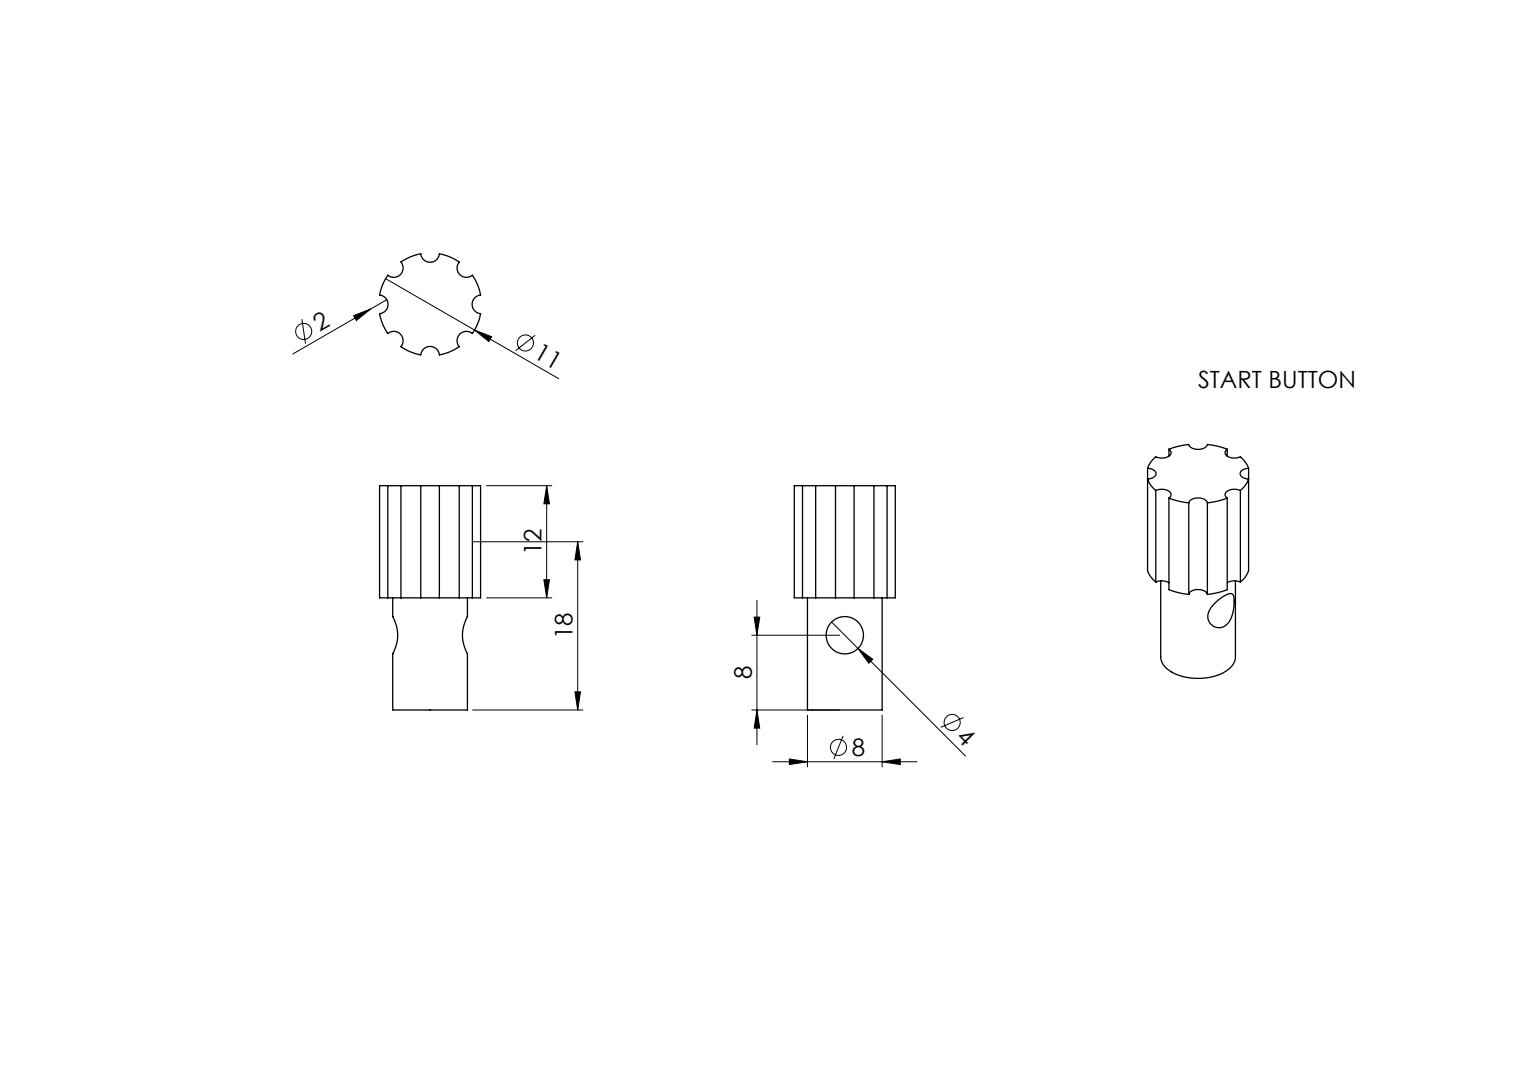
ISO-10303-21;
HEADER;
FILE_DESCRIPTION (('STEP AP214'),
    '1' );
FILE_NAME ('start button.step',
    '2026-10-26T11:20:31',
    ( '' ),
    ( '' ),
    'SwSTEP 2.0',
    'SolidWorks 2026',
    '' );
FILE_SCHEMA (( 'AUTOMOTIVE_DESIGN' ));
ENDSEC;

DATA;
#3=ORIENTED_EDGE ( 'NONE', *, *, #2058, .T. ) ;
#5=DIRECTION ( 'NONE',  ( 0.000000000000000000, 0.000000000000000000, 1.000000000000000000 ) ) ;
#6=ORIENTED_EDGE ( 'NONE', *, *, #2251, .T. ) ;
#8=ORIENTED_EDGE ( 'NONE', *, *, #613, .T. ) ;
#11=CARTESIAN_POINT ( 'NONE',  ( 3.575465955037824273, 33.89312899261130951, 7.205771075917312807 ) ) ;
#13=CARTESIAN_POINT ( 'NONE',  ( 3.900351855253538336, 31.20702153671021861, 9.895868398202676275 ) ) ;
#16=AXIS2_PLACEMENT_3D ( 'NONE', #2193, #1531, #438 ) ;
#20=AXIS2_PLACEMENT_3D ( 'NONE', #4406, #1830, #790 ) ;
#21=ORIENTED_EDGE ( 'NONE', *, *, #745, .T. ) ;
#25=CARTESIAN_POINT ( 'NONE',  ( -3.889087296526001047, 37.00000000000000000, 5.110912703473974084 ) ) ;
#26=DIRECTION ( 'NONE',  ( 0.000000000000000000, 0.000000000000000000, -1.000000000000000000 ) ) ;
#28=ORIENTED_EDGE ( 'NONE', *, *, #250, .F. ) ;
#35=APPLICATION_CONTEXT ( 'automotive_design' ) ;
#47=CARTESIAN_POINT ( 'NONE',  ( -3.606497132222527213, 31.99144327829980838, 10.73188315364928691 ) ) ;
#50=EDGE_CURVE ( 'NONE', #1185, #1168, #2904, .T. ) ;
#51=ORIENTED_EDGE ( 'NONE', *, *, #696, .F. ) ;
#52=VERTEX_POINT ( 'NONE', #2322 ) ;
#53=ORIENTED_EDGE ( 'NONE', *, *, #2142, .T. ) ;
#55=CIRCLE ( 'NONE', #1867, 1.000000000000000000 ) ;
#61=CARTESIAN_POINT ( 'NONE',  ( 3.120626071653185285, 37.00000000000000000, 4.471016347907789346 ) ) ;
#63=CIRCLE ( 'NONE', #1740, 4.000000000000000000 ) ;
#68=ADVANCED_FACE ( 'NONE', ( #4153 ), #1596, .T. ) ;
#73=CARTESIAN_POINT ( 'NONE',  ( -3.522877905629562711, 32.34829198493223146, 10.89542184998092367 ) ) ;
#76=EDGE_LOOP ( 'NONE', ( #1998, #356, #1571, #3856 ) ) ;
#84=EDGE_CURVE ( 'NONE', #2338, #1148, #4563, .T. ) ;
#86=EDGE_CURVE ( 'NONE', #3119, #3855, #2573, .T. ) ;
#94=LINE ( 'NONE', #3342, #4161 ) ;
#98=DIRECTION ( 'NONE',  ( 0.000000000000000000, 0.000000000000000000, 1.000000000000000000 ) ) ;
#103=EDGE_LOOP ( 'NONE', ( #598, #2944, #3052, #880 ) ) ;
#104=ORIENTED_EDGE ( 'NONE', *, *, #1011, .F. ) ;
#106=CARTESIAN_POINT ( 'NONE',  ( -3.889087296526001047, 37.00000000000000000, 5.110912703473974084 ) ) ;
#109=ORIENTED_EDGE ( 'NONE', *, *, #4683, .T. ) ;
#114=CARTESIAN_POINT ( 'NONE',  ( 2.255140518769849223E-14, 37.00000000000000000, 4.499999999999992895 ) ) ;
#116=CARTESIAN_POINT ( 'NONE',  ( -4.000043395258027878, 35.00008679053002680, 9.131973577465634762 ) ) ;
#120=CARTESIAN_POINT ( 'NONE',  ( 3.469446951953614189E-15, 37.00000000000000000, 8.999999999999992895 ) ) ;
#129=( GEOMETRIC_REPRESENTATION_CONTEXT ( 3 ) GLOBAL_UNCERTAINTY_ASSIGNED_CONTEXT ( ( #2638 ) ) GLOBAL_UNIT_ASSIGNED_CONTEXT ( ( #3790, #2760, #4527 ) ) REPRESENTATION_CONTEXT ( 'NONE', 'WORKASPACE' ) );
#133=DIRECTION ( 'NONE',  ( 0.000000000000000000, 0.000000000000000000, 1.000000000000000000 ) ) ;
#134=ORIENTED_EDGE ( 'NONE', *, *, #2569, .F. ) ;
#139=CARTESIAN_POINT ( 'NONE',  ( 2.255140518769849223E-14, 37.00000000000000000, 3.499999999999992895 ) ) ;
#141=CARTESIAN_POINT ( 'NONE',  ( -5.409090909090905619, 33.00000000000000000, 6.999999999999991118 ) ) ;
#145=CARTESIAN_POINT ( 'NONE',  ( 3.809567799457752368, 34.58652683892340463, 10.22463024623739081 ) ) ;
#154=SURFACE_STYLE_FILL_AREA ( #887 ) ;
#156=DIRECTION ( 'NONE',  ( 0.000000000000000000, 0.000000000000000000, 1.000000000000000000 ) ) ;
#158=DIRECTION ( 'NONE',  ( -0.000000000000000000, -1.000000000000000000, -0.000000000000000000 ) ) ;
#159=CARTESIAN_POINT ( 'NONE',  ( 3.120626071653123113, 37.00000000000000000, 13.52898365209223996 ) ) ;
#160=ORIENTED_EDGE ( 'NONE', *, *, #4437, .T. ) ;
#165=CARTESIAN_POINT ( 'NONE',  ( 3.967498225428659264, 34.93431228236265440, 8.474567154859101947 ) ) ;
#172=EDGE_LOOP ( 'NONE', ( #4370, #2757, #3708, #3979 ) ) ;
#178=LINE ( 'NONE', #2303, #3205 ) ;
#182=FACE_OUTER_BOUND ( 'NONE', #1092, .T. ) ;
#188=ORIENTED_EDGE ( 'NONE', *, *, #4683, .F. ) ;
#203=CARTESIAN_POINT ( 'NONE',  ( -3.889087296526055226, 49.00000000000000000, 12.88908729652595753 ) ) ;
#210=CARTESIAN_POINT ( 'NONE',  ( -3.464101615137750390, 33.00000000000000000, 6.999999999999991118 ) ) ;
#213=VERTEX_POINT ( 'NONE', #2094 ) ;
#215=EDGE_CURVE ( 'NONE', #3697, #378, #1086, .T. ) ;
#222=AXIS2_PLACEMENT_3D ( 'NONE', #601, #2758, #3141 ) ;
#223=ORIENTED_EDGE ( 'NONE', *, *, #3395, .T. ) ;
#231=CARTESIAN_POINT ( 'NONE',  ( -3.889087296526001047, 34.17157287525380838, 5.110912703473974084 ) ) ;
#233=VECTOR ( 'NONE', #4216, 1000.000000000000000 ) ;
#237=ORIENTED_EDGE ( 'NONE', *, *, #1871, .T. ) ;
#243=CIRCLE ( 'NONE', #3040, 1.000000000000000000 ) ;
#250=EDGE_CURVE ( 'NONE', #1339, #1902, #257, .T. ) ;
#253=EDGE_CURVE ( 'NONE', #1148, #1902, #1067, .T. ) ;
#257=LINE ( 'NONE', #3875, #233 ) ;
#264=AXIS2_PLACEMENT_3D ( 'NONE', #4299, #3243, #659 ) ;
#267=ADVANCED_FACE ( 'NONE', ( #621 ), #905, .F. ) ;
#269=DIRECTION ( 'NONE',  ( -0.000000000000000000, -1.000000000000000000, -0.000000000000000000 ) ) ;
#273=DIRECTION ( 'NONE',  ( 0.000000000000000000, 1.000000000000000000, 0.000000000000000000 ) ) ;
#277=VECTOR ( 'NONE', #1465, 1000.000000000000000 ) ;
#286=CARTESIAN_POINT ( 'NONE',  ( 3.469446951953614189E-15, 49.00000000000000000, 8.999999999999992895 ) ) ;
#291=AXIS2_PLACEMENT_3D ( 'NONE', #4539, #997, #2087 ) ;
#293=CARTESIAN_POINT ( 'NONE',  ( -3.120626071653146649, 43.00000000000000000, 4.471016347907768029 ) ) ;
#294=CIRCLE ( 'NONE', #1500, 1.000000000000000000 ) ;
#304=ORIENTED_EDGE ( 'NONE', *, *, #711, .T. ) ;
#306=CARTESIAN_POINT ( 'NONE',  ( 5.500000000000003553, 34.17157287525380838, 8.999999999999992895 ) ) ;
#307=VECTOR ( 'NONE', #4096, 1000.000000000000000 ) ;
#319=CARTESIAN_POINT ( 'NONE',  ( 3.993269581196953411, 31.01336414471273883, 8.733908321742495318 ) ) ;
#335=APPLICATION_CONTEXT ( 'automotive_design' ) ;
#341=DIRECTION ( 'NONE',  ( 1.000000000000000000, -0.000000000000000000, -0.000000000000000000 ) ) ;
#342=VECTOR ( 'NONE', #432, 1000.000000000000000 ) ;
#345=MECHANICAL_DESIGN_GEOMETRIC_PRESENTATION_REPRESENTATION('',(#2384),#129);
#356=ORIENTED_EDGE ( 'NONE', *, *, #4437, .F. ) ;
#358=CARTESIAN_POINT ( 'NONE',  ( 3.999885695961631793, 34.99977139185988051, 9.266511461428612151 ) ) ;
#359=CARTESIAN_POINT ( 'NONE',  ( -5.409090909090905619, 43.00000000000000000, 9.995859195463930646 ) ) ;
#361=CARTESIAN_POINT ( 'NONE',  ( 3.464101615137758383, 32.86534535152231484, 6.999999999999992006 ) ) ;
#366=CARTESIAN_POINT ( 'NONE',  ( 4.528983652092195555, 37.00000000000000000, 12.12062607165318973 ) ) ;
#367=AXIS2_PLACEMENT_3D ( 'NONE', #1611, #4592, #2382 ) ;
#371=ORIENTED_EDGE ( 'NONE', *, *, #2152, .T. ) ;
#377=VERTEX_POINT ( 'NONE', #3443 ) ;
#378=VERTEX_POINT ( 'NONE', #2133 ) ;
#391=CARTESIAN_POINT ( 'NONE',  ( -3.967441838779837582, 34.93419588968778555, 9.525690396061339271 ) ) ;
#393=VECTOR ( 'NONE', #632, 1000.000000000000000 ) ;
#395=EDGE_LOOP ( 'NONE', ( #4328, #2140, #4671, #3538 ) ) ;
#408=ORIENTED_EDGE ( 'NONE', *, *, #542, .F. ) ;
#411=CARTESIAN_POINT ( 'NONE',  ( 3.522982843720159796, 32.34803768106982602, 10.89519766348715102 ) ) ;
#412=CIRCLE ( 'NONE', #3674, 1.000000000000000000 ) ;
#415=CARTESIAN_POINT ( 'NONE',  ( -3.889087296526001047, 49.00000000000000000, 6.110912703473974084 ) ) ;
#432=DIRECTION ( 'NONE',  ( 0.000000000000000000, -1.000000000000000000, 0.000000000000000000 ) ) ;
#438=DIRECTION ( 'NONE',  ( 0.000000000000000000, 0.000000000000000000, 1.000000000000000000 ) ) ;
#439=CARTESIAN_POINT ( 'NONE',  ( -5.499999999999996447, 34.17157287525380838, 8.999999999999992895 ) ) ;
#441=CARTESIAN_POINT ( 'NONE',  ( -3.672134815396410179, 34.23001392835894308, 10.59780778022629377 ) ) ;
#445=CARTESIAN_POINT ( 'NONE',  ( -3.501495480098614443, 32.47366590808272235, 10.93402018205975601 ) ) ;
#446=CARTESIAN_POINT ( 'NONE',  ( 3.469446951953614189E-15, 49.00000000000000000, 8.999999999999992895 ) ) ;
#448=CARTESIAN_POINT ( 'NONE',  ( 3.469446951953614189E-15, 49.00000000000000000, 8.999999999999992895 ) ) ;
#451=AXIS2_PLACEMENT_3D ( 'NONE', #3078, #2717, #4317 ) ;
#460=VERTEX_POINT ( 'NONE', #3272 ) ;
#468=VERTEX_POINT ( 'NONE', #4017 ) ;
#479=DIRECTION ( 'NONE',  ( 0.000000000000000000, 1.000000000000000000, 0.000000000000000000 ) ) ;
#486=CARTESIAN_POINT ( 'NONE',  ( 3.601048973789312324, 31.98899025511026650, 10.74504312029988284 ) ) ;
#487=PRODUCT_DEFINITION ( 'UNKNOWN', '', #1349, #2416 ) ;
#494=CARTESIAN_POINT ( 'NONE',  ( 3.971780439164239063, 34.94497680528392891, 9.533653685786569909 ) ) ;
#497=DIRECTION ( 'NONE',  ( 0.000000000000000000, 0.000000000000000000, 1.000000000000000000 ) ) ;
#502=CARTESIAN_POINT ( 'NONE',  ( -3.120626071653146649, 49.00000000000000000, 4.471016347907768029 ) ) ;
#504=CARTESIAN_POINT ( 'NONE',  ( 4.528983652092238188, 37.00000000000000000, 5.879373928346857348 ) ) ;
#507=PRODUCT ( 'start button', 'start button', '', ( #1061 ) ) ;
#515=CARTESIAN_POINT ( 'NONE',  ( -3.889087296526001047, 34.17157287525380838, 6.110912703473974084 ) ) ;
#523=DIRECTION ( 'NONE',  ( 0.000000000000000000, 1.000000000000000000, -0.000000000000000000 ) ) ;
#525=VERTEX_POINT ( 'NONE', #3971 ) ;
#528=ORIENTED_EDGE ( 'NONE', *, *, #2213, .T. ) ;
#530=FACE_OUTER_BOUND ( 'NONE', #2627, .T. ) ;
#538=EDGE_CURVE ( 'NONE', #3343, #4108, #2239, .T. ) ;
#542=EDGE_CURVE ( 'NONE', #3343, #1490, #1089, .T. ) ;
#543=EDGE_CURVE ( 'NONE', #1651, #1279, #3319, .T. ) ;
#551=ORIENTED_EDGE ( 'NONE', *, *, #253, .F. ) ;
#558=CARTESIAN_POINT ( 'NONE',  ( 0.9958591954638854604, 37.00000000000000000, 14.40909090909091184 ) ) ;
#559=CARTESIAN_POINT ( 'NONE',  ( -4.528983652092210654, 49.00000000000000000, 5.879373928346826261 ) ) ;
#560=CARTESIAN_POINT ( 'NONE',  ( 5.409090909090911836, 37.00000000000000000, 8.004140804536053366 ) ) ;
#564=EDGE_CURVE ( 'NONE', #213, #2091, #3689, .T. ) ;
#565=CARTESIAN_POINT ( 'NONE',  ( 0.9958591954638856825, 49.00000000000000000, 14.40909090909091361 ) ) ;
#573=ORIENTED_EDGE ( 'NONE', *, *, #86, .F. ) ;
#574=VERTEX_POINT ( 'NONE', #3294 ) ;
#577=DIRECTION ( 'NONE',  ( 0.000000000000000000, 0.000000000000000000, -1.000000000000000000 ) ) ;
#581=DIRECTION ( 'NONE',  ( 0.000000000000000000, 0.000000000000000000, -1.000000000000000000 ) ) ;
#583=EDGE_CURVE ( 'NONE', #763, #2091, #94, .T. ) ;
#589=VECTOR ( 'NONE', #847, 1000.000000000000000 ) ;
#597=CARTESIAN_POINT ( 'NONE',  ( 3.889087296526035242, 49.00000000000000000, 5.110912703473999841 ) ) ;
#598=ORIENTED_EDGE ( 'NONE', *, *, #3273, .T. ) ;
#599=EDGE_LOOP ( 'NONE', ( #237, #2178, #2583, #28 ) ) ;
#601=CARTESIAN_POINT ( 'NONE',  ( 3.469446951953614189E-15, 49.00000000000000000, 8.999999999999992895 ) ) ;
#604=( NAMED_UNIT ( * ) SI_UNIT ( $, .STERADIAN. ) SOLID_ANGLE_UNIT ( ) );
#605=DIRECTION ( 'NONE',  ( -0.000000000000000000, 1.000000000000000000, -0.000000000000000000 ) ) ;
#608=LINE ( 'NONE', #3479, #393 ) ;
#610=DIRECTION ( 'NONE',  ( 0.000000000000000000, 0.000000000000000000, 1.000000000000000000 ) ) ;
#613=EDGE_CURVE ( 'NONE', #1651, #574, #4113, .T. ) ;
#621=FACE_OUTER_BOUND ( 'NONE', #395, .T. ) ;
#626=CARTESIAN_POINT ( 'NONE',  ( -0.9958591954639161026, 37.00000000000000000, 3.590909090909080170 ) ) ;
#628=DIRECTION ( 'NONE',  ( 0.000000000000000000, 0.000000000000000000, 1.000000000000000000 ) ) ;
#631=CIRCLE ( 'NONE', #2748, 5.500000000000000000 ) ;
#632=DIRECTION ( 'NONE',  ( -0.000000000000000000, 1.000000000000000000, -0.000000000000000000 ) ) ;
#646=ORIENTED_EDGE ( 'NONE', *, *, #4119, .F. ) ;
#653=CARTESIAN_POINT ( 'NONE',  ( 3.959305671612554781E-15, 43.00000000000000000, 12.99999999999999289 ) ) ;
#659=DIRECTION ( 'NONE',  ( 0.000000000000000000, -0.000000000000000000, 1.000000000000000000 ) ) ;
#666=CARTESIAN_POINT ( 'NONE',  ( -3.889087296526055226, 34.17157287525380838, 12.88908729652595753 ) ) ;
#670=FACE_OUTER_BOUND ( 'NONE', #858, .T. ) ;
#671=DIRECTION ( 'NONE',  ( -0.000000000000000000, -1.000000000000000000, -0.000000000000000000 ) ) ;
#675=ORIENTED_EDGE ( 'NONE', *, *, #4119, .T. ) ;
#683=CARTESIAN_POINT ( 'NONE',  ( 3.809991693235077026, 31.40492942523385267, 7.766500207085086593 ) ) ;
#692=AXIS2_PLACEMENT_3D ( 'NONE', #597, #3115, #4195 ) ;
#696=EDGE_CURVE ( 'NONE', #4356, #1339, #886, .T. ) ;
#709=FACE_BOUND ( 'NONE', #2678, .T. ) ;
#711=EDGE_CURVE ( 'NONE', #3855, #2686, #2311, .T. ) ;
#717=CARTESIAN_POINT ( 'NONE',  ( -5.409090909090905619, 33.00000000000000000, 10.99999999999999289 ) ) ;
#734=CARTESIAN_POINT ( 'NONE',  ( -3.523144759583856978, 33.65295909972188326, 7.105089090000585195 ) ) ;
#738=CARTESIAN_POINT ( 'NONE',  ( -3.575465955037816723, 32.10687100738867628, 7.205771075917310142 ) ) ;
#743=ORIENTED_EDGE ( 'NONE', *, *, #50, .F. ) ;
#745=EDGE_CURVE ( 'NONE', #378, #1543, #4609, .T. ) ;
#752=CARTESIAN_POINT ( 'NONE',  ( 3.501320667853366153, 32.47456368659583603, 10.93433813232663887 ) ) ;
#760=DIRECTION ( 'NONE',  ( 0.000000000000000000, 0.000000000000000000, 1.000000000000000000 ) ) ;
#763=VERTEX_POINT ( 'NONE', #565 ) ;
#764=ORIENTED_EDGE ( 'NONE', *, *, #2794, .T. ) ;
#782=CIRCLE ( 'NONE', #2359, 5.500000000000000000 ) ;
#783=ORIENTED_EDGE ( 'NONE', *, *, #925, .T. ) ;
#785=CARTESIAN_POINT ( 'NONE',  ( -3.706735793540070656, 31.67823920415836625, 7.493470964888215846 ) ) ;
#790=DIRECTION ( 'NONE',  ( 0.000000000000000000, -0.000000000000000000, 1.000000000000000000 ) ) ;
#801=DIRECTION ( 'NONE',  ( -0.000000000000000000, -1.000000000000000000, -0.000000000000000000 ) ) ;
#806=FACE_OUTER_BOUND ( 'NONE', #1194, .T. ) ;
#810=ORIENTED_EDGE ( 'NONE', *, *, #1129, .F. ) ;
#813=CARTESIAN_POINT ( 'NONE',  ( -5.409090909090905619, 33.00000000000000000, 8.999999999999992895 ) ) ;
#816=VERTEX_POINT ( 'NONE', #949 ) ;
#825=CARTESIAN_POINT ( 'NONE',  ( -3.775090262067420710, 34.50279623606592594, 10.32592777499123748 ) ) ;
#834=VERTEX_POINT ( 'NONE', #3943 ) ;
#842=EDGE_LOOP ( 'NONE', ( #3173, #371, #223, #2579 ) ) ;
#844=DIRECTION ( 'NONE',  ( 0.000000000000000000, -1.000000000000000000, 0.000000000000000000 ) ) ;
#845=CARTESIAN_POINT ( 'NONE',  ( 3.464101615137758827, 32.86736921533707800, 10.99999999999999822 ) ) ;
#847=DIRECTION ( 'NONE',  ( 1.000000000000000000, -0.000000000000000000, -0.000000000000000000 ) ) ;
#851=CARTESIAN_POINT ( 'NONE',  ( -3.889087296526001047, 37.00000000000000000, 6.110912703473974084 ) ) ;
#852=AXIS2_PLACEMENT_3D ( 'NONE', #4182, #2344, #156 ) ;
#854=CARTESIAN_POINT ( 'NONE',  ( 3.120626071653123557, 49.00000000000000000, 13.52898365209223996 ) ) ;
#857=EDGE_LOOP ( 'NONE', ( #3821, #3714, #2924, #2649 ) ) ;
#858=EDGE_LOOP ( 'NONE', ( #109, #134, #2567, #1803 ) ) ;
#870=AXIS2_PLACEMENT_3D ( 'NONE', #231, #973, #4564 ) ;
#872=VECTOR ( 'NONE', #2620, 1000.000000000000000 ) ;
#873=DIRECTION ( 'NONE',  ( -0.000000000000000000, 1.000000000000000000, -0.000000000000000000 ) ) ;
#874=CARTESIAN_POINT ( 'NONE',  ( 2.255140518769849223E-14, 49.00000000000000000, 3.499999999999992895 ) ) ;
#876=CARTESIAN_POINT ( 'NONE',  ( 3.672066530599467971, 34.22247196340288866, 10.58813356411693185 ) ) ;
#880=ORIENTED_EDGE ( 'NONE', *, *, #583, .T. ) ;
#881=ORIENTED_EDGE ( 'NONE', *, *, #3334, .F. ) ;
#886=CIRCLE ( 'NONE', #3466, 5.500000000000000000 ) ;
#887=FILL_AREA_STYLE ('',( #1690 ) ) ;
#889=CARTESIAN_POINT ( 'NONE',  ( 3.889087296526035242, 49.00000000000000000, 5.110912703473999841 ) ) ;
#905=CYLINDRICAL_SURFACE ( 'NONE', #367, 1.000000000000000000 ) ;
#917=( LENGTH_UNIT ( ) NAMED_UNIT ( * ) SI_UNIT ( .MILLI., .METRE. ) );
#922=CARTESIAN_POINT ( 'NONE',  ( -5.409090909090905619, 49.00000000000000000, 9.995859195463930646 ) ) ;
#924=EDGE_CURVE ( 'NONE', #816, #2965, #55, .T. ) ;
#925=EDGE_CURVE ( 'NONE', #1922, #378, #3566, .T. ) ;
#926=DIRECTION ( 'NONE',  ( 0.000000000000000000, 0.000000000000000000, -1.000000000000000000 ) ) ;
#934=ORIENTED_EDGE ( 'NONE', *, *, #3848, .F. ) ;
#936=DIRECTION ( 'NONE',  ( 0.000000000000000000, 1.000000000000000000, 0.000000000000000000 ) ) ;
#938=FACE_OUTER_BOUND ( 'NONE', #842, .T. ) ;
#939=B_SPLINE_CURVE_WITH_KNOTS ( 'NONE', 3,
 ( #3550, #361, #4320, #3942, #4662, #2626, #1434, #683, #1814, #2127, #1391, #319, #1769, #3219, #4687, #1060, #3265, #13, #1456, #1108, #3645, #2237, #486, #411, #752, #3006, #845, #4435 ),
 .UNSPECIFIED., .F., .F.,
 ( 4, 2, 2, 2, 2, 2, 2, 2, 2, 2, 2, 2, 2, 4 ),
 ( 0.000000000000000000, 0.0003975746136738169344, 0.0007951492273476338688, 0.001590298454695268605, 0.002385447682042902799, 0.002783022295716720655, 0.003180596909390538511, 0.003578171523064356367, 0.003975746136738174223, 0.004373320750411992079, 0.004770895364085809068, 0.005566044591433457790, 0.005963619205107282585, 0.006361193818781106513 ),
 .UNSPECIFIED. ) ;
#940=FACE_OUTER_BOUND ( 'NONE', #970, .T. ) ;
#941=VECTOR ( 'NONE', #269, 1000.000000000000000 ) ;
#942=ORIENTED_EDGE ( 'NONE', *, *, #2058, .F. ) ;
#949=CARTESIAN_POINT ( 'NONE',  ( 3.889087296526035242, 37.00000000000000000, 6.110912703473999841 ) ) ;
#961=CYLINDRICAL_SURFACE ( 'NONE', #2888, 5.500000000000000000 ) ;
#963=B_SPLINE_CURVE_WITH_KNOTS ( 'NONE', 3,
 ( #3619, #2631, #2268, #2675, #1974, #1608, #1899, #876, #2247, #4140, #145, #2313, #4359, #494, #358, #3781, #1585, #165, #2291, #3061, #4516, #1103, #3983, #1809, #11, #1451, #1949, #4094, #3370, #2907 ),
 .UNSPECIFIED., .F., .F.,
 ( 4, 2, 2, 2, 2, 2, 2, 2, 2, 2, 2, 2, 2, 2, 4 ),
 ( 0.006361193818781106513, 0.006758065648931968657, 0.007154937479082830801, 0.007551809309233692945, 0.007948681139384555089, 0.008345552969535416366, 0.008742424799686279377, 0.009536168459987998461, 0.009933040290138858003, 0.01032991212028971928, 0.01112365578059143836, 0.01152052761074228923, 0.01191739944089314357, 0.01231427127104399617, 0.01271114310119484878 ),
 .UNSPECIFIED. ) ;
#964=FACE_OUTER_BOUND ( 'NONE', #1217, .T. ) ;
#967=( NAMED_UNIT ( * ) PLANE_ANGLE_UNIT ( ) SI_UNIT ( $, .RADIAN. ) );
#970=EDGE_LOOP ( 'NONE', ( #3118, #2045, #646, #4146 ) ) ;
#973=DIRECTION ( 'NONE',  ( -0.000000000000000000, 1.000000000000000000, -0.000000000000000000 ) ) ;
#986=DIRECTION ( 'NONE',  ( 0.000000000000000000, 1.000000000000000000, 0.000000000000000000 ) ) ;
#997=DIRECTION ( 'NONE',  ( 0.000000000000000000, 1.000000000000000000, 0.000000000000000000 ) ) ;
#1007=DIRECTION ( 'NONE',  ( 0.000000000000000000, 0.000000000000000000, 1.000000000000000000 ) ) ;
#1011=EDGE_CURVE ( 'NONE', #1930, #2608, #4613, .T. ) ;
#1012=ADVANCED_FACE ( 'NONE', ( #1758, #3611 ), #1380, .T. ) ;
#1013=DIRECTION ( 'NONE',  ( 0.000000000000000000, 0.000000000000000000, 1.000000000000000000 ) ) ;
#1019=CARTESIAN_POINT ( 'NONE',  ( -3.967457472430134580, 34.93422823600056404, 8.474369013652145455 ) ) ;
#1022=CIRCLE ( 'NONE', #1936, 1.000000000000000888 ) ;
#1044=CARTESIAN_POINT ( 'NONE',  ( 3.469446951953614189E-15, 43.00000000000000000, 8.999999999999992895 ) ) ;
#1051=CARTESIAN_POINT ( 'NONE',  ( 2.255140518769849223E-14, 34.17157287525380838, 4.499999999999992895 ) ) ;
#1056=CARTESIAN_POINT ( 'NONE',  ( 3.469446951953614189E-15, 37.00000000000000000, 8.999999999999992895 ) ) ;
#1060=CARTESIAN_POINT ( 'NONE',  ( 3.967441838779844687, 31.06580411031222866, 9.525690396061342824 ) ) ;
#1061=PRODUCT_CONTEXT ( 'NONE', #335, 'mechanical' ) ;
#1066=EDGE_CURVE ( 'NONE', #3374, #1168, #4164, .T. ) ;
#1067=CIRCLE ( 'NONE', #692, 0.9999999999999997780 ) ;
#1068=EDGE_LOOP ( 'NONE', ( #104, #3039, #764, #2252 ) ) ;
#1072=CIRCLE ( 'NONE', #3965, 5.500000000000000000 ) ;
#1075=CARTESIAN_POINT ( 'NONE',  ( 5.500000000000003553, 49.00000000000000000, 8.999999999999992895 ) ) ;
#1078=DIRECTION ( 'NONE',  ( 0.000000000000000000, 0.000000000000000000, 1.000000000000000000 ) ) ;
#1082=CYLINDRICAL_SURFACE ( 'NONE', #4184, 2.000000000000000888 ) ;
#1086=CIRCLE ( 'NONE', #3744, 1.000000000000000000 ) ;
#1089=LINE ( 'NONE', #2524, #2622 ) ;
#1090=ORIENTED_EDGE ( 'NONE', *, *, #4551, .T. ) ;
#1092=EDGE_LOOP ( 'NONE', ( #934, #1967, #4570, #1475 ) ) ;
#1097=EDGE_LOOP ( 'NONE', ( #4260, #810, #1357, #2559 ) ) ;
#1100=ADVANCED_FACE ( 'NONE', ( #1926 ), #4450, .F. ) ;
#1103=CARTESIAN_POINT ( 'NONE',  ( 3.706735793540077761, 34.32176079584164086, 7.493470964888216734 ) ) ;
#1105=EDGE_LOOP ( 'NONE', ( #2628, #1291, #1658, #3274 ) ) ;
#1108=CARTESIAN_POINT ( 'NONE',  ( 3.809422024637068471, 31.41382050535269954, 10.22508852591141348 ) ) ;
#1111=COLOUR_RGB ( '',0.8941176470588234615, 0.8941176470588234615, 0.8941176470588234615 ) ;
#1120=CARTESIAN_POINT ( 'NONE',  ( -3.472185852622982516, 32.73050154287725633, 7.013837769849707193 ) ) ;
#1124=ORIENTED_EDGE ( 'NONE', *, *, #2983, .F. ) ;
#1129=EDGE_CURVE ( 'NONE', #1185, #1877, #4475, .T. ) ;
#1136=CIRCLE ( 'NONE', #2119, 5.500000000000000000 ) ;
#1148=VERTEX_POINT ( 'NONE', #3751 ) ;
#1160=CARTESIAN_POINT ( 'NONE',  ( -3.900351855253532118, 34.79297846328978494, 9.895868398202676275 ) ) ;
#1163=CARTESIAN_POINT ( 'NONE',  ( -3.900821110013151127, 31.20601586925484128, 9.893616917921782772 ) ) ;
#1165=CARTESIAN_POINT ( 'NONE',  ( 5.409090909090912724, 49.00000000000000000, 9.995859195463930646 ) ) ;
#1166=ORIENTED_EDGE ( 'NONE', *, *, #4352, .T. ) ;
#1168=VERTEX_POINT ( 'NONE', #1165 ) ;
#1185=VERTEX_POINT ( 'NONE', #3678 ) ;
#1186=CARTESIAN_POINT ( 'NONE',  ( -3.993355759804213090, 31.01319048188283034, 8.734987511292612083 ) ) ;
#1192=VERTEX_POINT ( 'NONE', #854 ) ;
#1194=EDGE_LOOP ( 'NONE', ( #1868, #3653, #4355, #573, #2187, #3019, #2155, #2363, #675, #1469, #528, #3426, #2410, #1223, #1903, #551, #1462, #3424, #3203 ) ) ;
#1196=CARTESIAN_POINT ( 'NONE',  ( 5.409090909090912724, 43.00000000000000000, 8.004140804536053366 ) ) ;
#1198=LINE ( 'NONE', #3735, #3004 ) ;
#1199=VERTEX_POINT ( 'NONE', #4495 ) ;
#1217=EDGE_LOOP ( 'NONE', ( #1166, #783, #21, #1124 ) ) ;
#1220=CARTESIAN_POINT ( 'NONE',  ( 3.469446951953614189E-15, 37.00000000000000000, 8.999999999999992895 ) ) ;
#1223=ORIENTED_EDGE ( 'NONE', *, *, #1066, .F. ) ;
#1231=CARTESIAN_POINT ( 'NONE',  ( -3.501320667853359048, 33.52543631340415686, 10.93433813232664242 ) ) ;
#1232=VECTOR ( 'NONE', #2851, 1000.000000000000000 ) ;
#1240=EDGE_CURVE ( 'NONE', #3697, #2686, #1072, .T. ) ;
#1247=SURFACE_STYLE_USAGE ( .BOTH. , #1594 ) ;
#1248=DIRECTION ( 'NONE',  ( 0.000000000000000000, 0.000000000000000000, -1.000000000000000000 ) ) ;
#1251=DIRECTION ( 'NONE',  ( -0.000000000000000000, -1.000000000000000000, -0.000000000000000000 ) ) ;
#1254=DIRECTION ( 'NONE',  ( 0.000000000000000000, 1.000000000000000000, 0.000000000000000000 ) ) ;
#1256=VECTOR ( 'NONE', #4088, 1000.000000000000000 ) ;
#1264=EDGE_CURVE ( 'NONE', #468, #4108, #2711, .T. ) ;
#1267=EDGE_LOOP ( 'NONE', ( #4285, #6, #743, #3830 ) ) ;
#1279=VERTEX_POINT ( 'NONE', #4525 ) ;
#1291=ORIENTED_EDGE ( 'NONE', *, *, #1386, .T. ) ;
#1293=ORIENTED_EDGE ( 'NONE', *, *, #4352, .F. ) ;
#1302=DIRECTION ( 'NONE',  ( 0.7071067811865392461, 0.000000000000000000, 0.7071067811865557884 ) ) ;
#1322=CARTESIAN_POINT ( 'NONE',  ( -3.889087296526001047, 49.00000000000000000, 5.110912703473974084 ) ) ;
#1328=DIRECTION ( 'NONE',  ( 0.000000000000000000, 0.000000000000000000, 1.000000000000000000 ) ) ;
#1339=VERTEX_POINT ( 'NONE', #504 ) ;
#1340=CARTESIAN_POINT ( 'NONE',  ( 3.469446951953614189E-15, 25.00000000000000000, 8.999999999999992895 ) ) ;
#1341=DIRECTION ( 'NONE',  ( -0.000000000000000000, -1.000000000000000000, -0.000000000000000000 ) ) ;
#1349=PRODUCT_DEFINITION_FORMATION_WITH_SPECIFIED_SOURCE ( 'ANY', '', #507, .NOT_KNOWN. ) ;
#1352=CARTESIAN_POINT ( 'NONE',  ( 3.469446951953614189E-15, 49.00000000000000000, 8.999999999999992895 ) ) ;
#1357=ORIENTED_EDGE ( 'NONE', *, *, #3888, .T. ) ;
#1362=ADVANCED_FACE ( 'NONE', ( #938 ), #961, .T. ) ;
#1364=CARTESIAN_POINT ( 'NONE',  ( 3.469446951953614189E-15, 49.00000000000000000, 8.999999999999992895 ) ) ;
#1373=FACE_OUTER_BOUND ( 'NONE', #857, .T. ) ;
#1374=CARTESIAN_POINT ( 'NONE',  ( -3.876963039844159020, 34.74320821126782732, 7.985516166298877394 ) ) ;
#1380=CYLINDRICAL_SURFACE ( 'NONE', #2470, 4.000000000000000000 ) ;
#1385=DIRECTION ( 'NONE',  ( 0.000000000000000000, 0.000000000000000000, 1.000000000000000000 ) ) ;
#1386=EDGE_CURVE ( 'NONE', #1279, #1199, #3610, .T. ) ;
#1387=DIRECTION ( 'NONE',  ( -0.000000000000000000, 1.000000000000000000, -0.000000000000000000 ) ) ;
#1391=CARTESIAN_POINT ( 'NONE',  ( 3.967457472430142573, 31.06577176399945017, 8.474369013652145455 ) ) ;
#1400=CARTESIAN_POINT ( 'NONE',  ( 3.889087296526035242, 34.17157287525380838, 6.110912703473999841 ) ) ;
#1402=DIRECTION ( 'NONE',  ( -0.000000000000000000, 1.000000000000000000, -0.000000000000000000 ) ) ;
#1411=FACE_OUTER_BOUND ( 'NONE', #3680, .T. ) ;
#1420=DIRECTION ( 'NONE',  ( -0.000000000000000000, 1.000000000000000000, 0.000000000000000000 ) ) ;
#1422=ORIENTED_EDGE ( 'NONE', *, *, #1264, .F. ) ;
#1425=DIRECTION ( 'NONE',  ( 0.000000000000000000, 1.000000000000000000, 0.000000000000000000 ) ) ;
#1430=DIRECTION ( 'NONE',  ( 0.000000000000000000, 1.000000000000000000, 0.000000000000000000 ) ) ;
#1432=AXIS2_PLACEMENT_3D ( 'NONE', #1352, #1675, #3152 ) ;
#1433=LINE ( 'NONE', #2594, #1810 ) ;
#1434=CARTESIAN_POINT ( 'NONE',  ( 3.672900200782976743, 31.76776247384029972, 7.403954086897937437 ) ) ;
#1437=CARTESIAN_POINT ( 'NONE',  ( -0.9958591954639161026, 49.00000000000000000, 3.590909090909080170 ) ) ;
#1438=ADVANCED_FACE ( 'NONE', ( #1777 ), #1735, .T. ) ;
#1440=EDGE_CURVE ( 'NONE', #816, #1148, #2412, .T. ) ;
#1447=EDGE_LOOP ( 'NONE', ( #2183, #2534, #3731, #160 ) ) ;
#1450=CARTESIAN_POINT ( 'NONE',  ( -5.499999999999996447, 37.00000000000000000, 8.999999999999992895 ) ) ;
#1451=CARTESIAN_POINT ( 'NONE',  ( 3.523178763948789705, 33.65307825300501321, 7.105158153061387871 ) ) ;
#1456=CARTESIAN_POINT ( 'NONE',  ( 3.871991356174931731, 31.26893492619631942, 10.01005989714294664 ) ) ;
#1457=SHAPE_DEFINITION_REPRESENTATION ( #4494, #3382 ) ;
#1459=CYLINDRICAL_SURFACE ( 'NONE', #4138, 1.000000000000000888 ) ;
#1462=ORIENTED_EDGE ( 'NONE', *, *, #84, .F. ) ;
#1463=CARTESIAN_POINT ( 'NONE',  ( -3.775946040281024541, 31.49506148730309008, 10.32350191120198346 ) ) ;
#1465=DIRECTION ( 'NONE',  ( -0.000000000000000000, 1.000000000000000000, -0.000000000000000000 ) ) ;
#1467=AXIS2_PLACEMENT_3D ( 'NONE', #2402, #3508, #4585 ) ;
#1469=ORIENTED_EDGE ( 'NONE', *, *, #3532, .F. ) ;
#1470=DIRECTION ( 'NONE',  ( 0.000000000000000000, 1.000000000000000000, 0.000000000000000000 ) ) ;
#1475=ORIENTED_EDGE ( 'NONE', *, *, #86, .T. ) ;
#1478=CARTESIAN_POINT ( 'NONE',  ( -0.9958591954639913757, 43.00000000000000000, 14.40909090909089230 ) ) ;
#1485=VERTEX_POINT ( 'NONE', #626 ) ;
#1487=CARTESIAN_POINT ( 'NONE',  ( -3.809567799457745263, 31.41347316107661314, 10.22463024623739081 ) ) ;
#1490=VERTEX_POINT ( 'NONE', #3517 ) ;
#1492=EDGE_LOOP ( 'NONE', ( #3105, #3631 ) ) ;
#1493=CARTESIAN_POINT ( 'NONE',  ( 3.120626071653123113, 43.00000000000000000, 13.52898365209223996 ) ) ;
#1500=AXIS2_PLACEMENT_3D ( 'NONE', #106, #1546, #2298 ) ;
#1502=MECHANICAL_DESIGN_GEOMETRIC_PRESENTATION_REPRESENTATION('',(#2330),#3637);
#1505=AXIS2_PLACEMENT_3D ( 'NONE', #1056, #3963, #610 ) ;
#1510=CYLINDRICAL_SURFACE ( 'NONE', #2136, 5.500000000000000000 ) ;
#1516=DIRECTION ( 'NONE',  ( 0.000000000000000000, 0.000000000000000000, 1.000000000000000000 ) ) ;
#1525=FACE_OUTER_BOUND ( 'NONE', #1105, .T. ) ;
#1531=DIRECTION ( 'NONE',  ( -0.000000000000000000, -1.000000000000000000, -0.000000000000000000 ) ) ;
#1532=FACE_OUTER_BOUND ( 'NONE', #76, .T. ) ;
#1533=DIRECTION ( 'NONE',  ( 0.000000000000000000, -1.000000000000000000, -0.000000000000000000 ) ) ;
#1534=AXIS2_PLACEMENT_3D ( 'NONE', #4579, #4267, #1007 ) ;
#1538=DIRECTION ( 'NONE',  ( 0.000000000000000000, 1.000000000000000000, 0.000000000000000000 ) ) ;
#1540=DIRECTION ( 'NONE',  ( 0.000000000000000000, 1.000000000000000000, 0.000000000000000000 ) ) ;
#1543=VERTEX_POINT ( 'NONE', #2967 ) ;
#1546=DIRECTION ( 'NONE',  ( -0.000000000000000000, -1.000000000000000000, -0.000000000000000000 ) ) ;
#1556=EDGE_CURVE ( 'NONE', #1279, #1651, #3779, .T. ) ;
#1557=LINE ( 'NONE', #515, #1256 ) ;
#1558=CARTESIAN_POINT ( 'NONE',  ( -3.471741185006985919, 33.26424185130363043, 10.98693824102217498 ) ) ;
#1561=EDGE_CURVE ( 'NONE', #3402, #52, #243, .T. ) ;
#1568=ORIENTED_EDGE ( 'NONE', *, *, #2355, .F. ) ;
#1571=ORIENTED_EDGE ( 'NONE', *, *, #2927, .T. ) ;
#1578=DIRECTION ( 'NONE',  ( -0.000000000000000000, -1.000000000000000000, -0.000000000000000000 ) ) ;
#1580=ADVANCED_FACE ( 'NONE', ( #3654 ), #1510, .T. ) ;
#1581=DIRECTION ( 'NONE',  ( 0.000000000000000000, 0.000000000000000000, 1.000000000000000000 ) ) ;
#1585=CARTESIAN_POINT ( 'NONE',  ( 3.993355759804221083, 34.98680951811717676, 8.734987511292612083 ) ) ;
#1592=DIRECTION ( 'NONE',  ( 0.000000000000000000, -1.000000000000000000, 0.000000000000000000 ) ) ;
#1594=SURFACE_SIDE_STYLE ('',( #154 ) ) ;
#1596=CYLINDRICAL_SURFACE ( 'NONE', #4640, 5.500000000000000000 ) ;
#1599=DIRECTION ( 'NONE',  ( 0.000000000000000000, 0.000000000000000000, -1.000000000000000000 ) ) ;
#1608=CARTESIAN_POINT ( 'NONE',  ( 3.575798854573977614, 33.89464632526108545, 10.79358726550606029 ) ) ;
#1611=CARTESIAN_POINT ( 'NONE',  ( 3.889087296526035242, 34.17157287525380838, 5.110912703473999841 ) ) ;
#1612=ORIENTED_EDGE ( 'NONE', *, *, #3207, .T. ) ;
#1615=EDGE_LOOP ( 'NONE', ( #3368, #3959, #2654, #1090 ) ) ;
#1623=LINE ( 'NONE', #4462, #2436 ) ;
#1624=CYLINDRICAL_SURFACE ( 'NONE', #451, 5.500000000000000000 ) ;
#1635=ORIENTED_EDGE ( 'NONE', *, *, #3271, .F. ) ;
#1637=ORIENTED_EDGE ( 'NONE', *, *, #1561, .F. ) ;
#1641=PRESENTATION_STYLE_ASSIGNMENT (( #1247 ) ) ;
#1651=VERTEX_POINT ( 'NONE', #210 ) ;
#1658=ORIENTED_EDGE ( 'NONE', *, *, #4037, .F. ) ;
#1659=EDGE_LOOP ( 'NONE', ( #4477, #4218 ) ) ;
#1672=DIRECTION ( 'NONE',  ( 0.000000000000000000, 0.000000000000000000, 1.000000000000000000 ) ) ;
#1675=DIRECTION ( 'NONE',  ( -0.000000000000000000, -1.000000000000000000, -0.000000000000000000 ) ) ;
#1678=DIRECTION ( 'NONE',  ( 0.000000000000000000, 1.000000000000000000, 0.000000000000000000 ) ) ;
#1690=FILL_AREA_STYLE_COLOUR ( '', #1111 ) ;
#1693=FACE_OUTER_BOUND ( 'NONE', #172, .T. ) ;
#1711=DIRECTION ( 'NONE',  ( 1.000000000000000000, -0.000000000000000000, -0.000000000000000000 ) ) ;
#1712=DIRECTION ( 'NONE',  ( 0.000000000000000000, 0.000000000000000000, 1.000000000000000000 ) ) ;
#1721=DIRECTION ( 'NONE',  ( 0.000000000000000000, 0.000000000000000000, 1.000000000000000000 ) ) ;
#1728=CARTESIAN_POINT ( 'NONE',  ( -3.601840573626707176, 34.01414095348192035, 7.256529352857233661 ) ) ;
#1732=AXIS2_PLACEMENT_3D ( 'NONE', #1853, #1470, #3617 ) ;
#1735=CYLINDRICAL_SURFACE ( 'NONE', #4489, 5.500000000000000000 ) ;
#1740=AXIS2_PLACEMENT_3D ( 'NONE', #3238, #1430, #2441 ) ;
#1750=ADVANCED_FACE ( 'NONE', ( #3579, #2845 ), #4304, .T. ) ;
#1757=CARTESIAN_POINT ( 'NONE',  ( 5.500000000000003553, 37.00000000000000000, 8.999999999999992895 ) ) ;
#1758=FACE_OUTER_BOUND ( 'NONE', #3994, .T. ) ;
#1769=CARTESIAN_POINT ( 'NONE',  ( 3.999956176514755768, 31.00008764698453945, 8.865408859660238505 ) ) ;
#1774=ORIENTED_EDGE ( 'NONE', *, *, #3561, .F. ) ;
#1777=FACE_OUTER_BOUND ( 'NONE', #103, .T. ) ;
#1780=CARTESIAN_POINT ( 'NONE',  ( 0.000000000000000000, 0.000000000000000000, 0.000000000000000000 ) ) ;
#1784=AXIS2_PLACEMENT_3D ( 'NONE', #3902, #1402, #4698 ) ;
#1791=AXIS2_PLACEMENT_3D ( 'NONE', #3356, #479, #1516 ) ;
#1792=AXIS2_PLACEMENT_3D ( 'NONE', #874, #2725, #2061 ) ;
#1803=ORIENTED_EDGE ( 'NONE', *, *, #2251, .F. ) ;
#1809=CARTESIAN_POINT ( 'NONE',  ( 3.606676218660111122, 34.00918236503840575, 7.268492701228249864 ) ) ;
#1810=VECTOR ( 'NONE', #3966, 1000.000000000000000 ) ;
#1814=CARTESIAN_POINT ( 'NONE',  ( 3.876963039844164793, 31.25679178873219044, 7.985516166298875618 ) ) ;
#1818=CARTESIAN_POINT ( 'NONE',  ( 3.469446951953614189E-15, 37.00000000000000000, 8.999999999999992895 ) ) ;
#1830=DIRECTION ( 'NONE',  ( 0.000000000000000000, 1.000000000000000000, 0.000000000000000000 ) ) ;
#1833=VECTOR ( 'NONE', #1711, 1000.000000000000000 ) ;
#1853=CARTESIAN_POINT ( 'NONE',  ( 3.469446951953614189E-15, 37.00000000000000000, 8.999999999999992895 ) ) ;
#1859=AXIS2_PLACEMENT_3D ( 'NONE', #1757, #3209, #628 ) ;
#1862=AXIS2_PLACEMENT_3D ( 'NONE', #4065, #801, #2672 ) ;
#1865=CARTESIAN_POINT ( 'NONE',  ( -3.464101615137750390, 33.00000000000000000, 10.99999999999999467 ) ) ;
#1867=AXIS2_PLACEMENT_3D ( 'NONE', #4432, #2616, #3590 ) ;
#1868=ORIENTED_EDGE ( 'NONE', *, *, #215, .F. ) ;
#1871=EDGE_CURVE ( 'NONE', #1339, #816, #3820, .T. ) ;
#1877=VERTEX_POINT ( 'NONE', #366 ) ;
#1899=CARTESIAN_POINT ( 'NONE',  ( 3.606497132222534319, 34.00855672170019517, 10.73188315364928513 ) ) ;
#1902=VERTEX_POINT ( 'NONE', #3315 ) ;
#1903=ORIENTED_EDGE ( 'NONE', *, *, #2884, .T. ) ;
#1922=VERTEX_POINT ( 'NONE', #114 ) ;
#1926=FACE_OUTER_BOUND ( 'NONE', #1097, .T. ) ;
#1930=VERTEX_POINT ( 'NONE', #3719 ) ;
#1936=AXIS2_PLACEMENT_3D ( 'NONE', #2015, #3468, #2381 ) ;
#1943=CIRCLE ( 'NONE', #1859, 0.9999999999999991118 ) ;
#1949=CARTESIAN_POINT ( 'NONE',  ( 3.501826698183293729, 33.52853102779839389, 7.066576927953558851 ) ) ;
#1954=ORIENTED_EDGE ( 'NONE', *, *, #543, .F. ) ;
#1958=ADVANCED_FACE ( 'NONE', ( #3641 ), #2229, .F. ) ;
#1961=( LENGTH_UNIT ( ) NAMED_UNIT ( * ) SI_UNIT ( .MILLI., .METRE. ) );
#1965=CARTESIAN_POINT ( 'NONE',  ( 3.469446951953614189E-15, 25.00000000000000000, 8.999999999999992895 ) ) ;
#1967=ORIENTED_EDGE ( 'NONE', *, *, #1561, .T. ) ;
#1968=VECTOR ( 'NONE', #2952, 1000.000000000000000 ) ;
#1974=CARTESIAN_POINT ( 'NONE',  ( 3.522877905629569817, 33.65170801506776854, 10.89542184998092189 ) ) ;
#1991=CLOSED_SHELL ( 'NONE', ( #3008, #4653, #4700, #3304, #1750, #3991, #3108, #1580, #3130, #1438, #4562, #68, #1362, #1012, #1958, #2897, #3358, #3740, #3863, #3623, #2350, #1100, #2865, #267, #3737, #2562 ) ) ;
#1996=ADVANCED_BREP_SHAPE_REPRESENTATION ( '', ( #3033, #2928 ), #3388 ) ;
#1998=ORIENTED_EDGE ( 'NONE', *, *, #2429, .T. ) ;
#2007=DIRECTION ( 'NONE',  ( 0.000000000000000000, 1.000000000000000000, 0.000000000000000000 ) ) ;
#2010=CIRCLE ( 'NONE', #3076, 5.500000000000000000 ) ;
#2015=CARTESIAN_POINT ( 'NONE',  ( 3.889087296525981063, 37.00000000000000000, 12.88908729652603746 ) ) ;
#2045=ORIENTED_EDGE ( 'NONE', *, *, #4098, .T. ) ;
#2051=DIRECTION ( 'NONE',  ( -0.7071067811865437980, 0.000000000000000000, -0.7071067811865512365 ) ) ;
#2058=EDGE_CURVE ( 'NONE', #52, #3445, #631, .T. ) ;
#2061=DIRECTION ( 'NONE',  ( -1.000000000000000000, 0.000000000000000000, -3.469446951953614189E-15 ) ) ;
#2087=DIRECTION ( 'NONE',  ( 1.000000000000000000, 0.000000000000000000, 1.040834085586084257E-14 ) ) ;
#2091=VERTEX_POINT ( 'NONE', #558 ) ;
#2093=EDGE_LOOP ( 'NONE', ( #4291, #3164 ) ) ;
#2094=CARTESIAN_POINT ( 'NONE',  ( -0.9958591954639911537, 37.00000000000000000, 14.40909090909089052 ) ) ;
#2098=CARTESIAN_POINT ( 'NONE',  ( 3.469446951953614189E-15, 25.00000000000000000, 4.999999999999992006 ) ) ;
#2108=AXIS2_PLACEMENT_3D ( 'NONE', #446, #1538, #2991 ) ;
#2114=VECTOR ( 'NONE', #1592, 1000.000000000000000 ) ;
#2117=DIRECTION ( 'NONE',  ( -0.000000000000000000, -1.000000000000000000, -0.000000000000000000 ) ) ;
#2119=AXIS2_PLACEMENT_3D ( 'NONE', #4251, #4684, #1328 ) ;
#2127=CARTESIAN_POINT ( 'NONE',  ( 3.948082828799474697, 31.10544434314014239, 8.346052798592717537 ) ) ;
#2130=AXIS2_PLACEMENT_3D ( 'NONE', #3371, #523, #497 ) ;
#2133=CARTESIAN_POINT ( 'NONE',  ( 2.255140518769849223E-14, 49.00000000000000000, 4.499999999999992895 ) ) ;
#2136=AXIS2_PLACEMENT_3D ( 'NONE', #4421, #2606, #926 ) ;
#2140=ORIENTED_EDGE ( 'NONE', *, *, #924, .T. ) ;
#2142=EDGE_CURVE ( 'NONE', #3119, #52, #178, .T. ) ;
#2152=EDGE_CURVE ( 'NONE', #3697, #1485, #1623, .T. ) ;
#2154=CARTESIAN_POINT ( 'NONE',  ( -3.464101615137750390, 33.00000000000000000, 6.999999999999991118 ) ) ;
#2155=ORIENTED_EDGE ( 'NONE', *, *, #2586, .T. ) ;
#2160=CARTESIAN_POINT ( 'NONE',  ( 3.469446951953614189E-15, 37.00000000000000000, 8.999999999999992895 ) ) ;
#2172=FACE_OUTER_BOUND ( 'NONE', #4701, .T. ) ;
#2178=ORIENTED_EDGE ( 'NONE', *, *, #1440, .T. ) ;
#2179=CARTESIAN_POINT ( 'NONE',  ( -3.971780439164231513, 31.05502319471607819, 9.533653685786568133 ) ) ;
#2180=DIRECTION ( 'NONE',  ( 0.000000000000000000, 1.000000000000000000, 0.000000000000000000 ) ) ;
#2182=ORIENTED_EDGE ( 'NONE', *, *, #2884, .F. ) ;
#2183=ORIENTED_EDGE ( 'NONE', *, *, #2475, .T. ) ;
#2185=DIRECTION ( 'NONE',  ( -0.000000000000000000, -1.000000000000000000, -0.000000000000000000 ) ) ;
#2187=ORIENTED_EDGE ( 'NONE', *, *, #2781, .T. ) ;
#2190=DIRECTION ( 'NONE',  ( 0.000000000000000000, 1.000000000000000000, 0.000000000000000000 ) ) ;
#2193=CARTESIAN_POINT ( 'NONE',  ( 3.889087296526035242, 37.00000000000000000, 5.110912703473999841 ) ) ;
#2195=CARTESIAN_POINT ( 'NONE',  ( -3.522982843720154467, 33.65196231893016687, 10.89519766348715457 ) ) ;
#2204=LINE ( 'NONE', #1493, #1968 ) ;
#2213=EDGE_CURVE ( 'NONE', #763, #1192, #782, .T. ) ;
#2221=CARTESIAN_POINT ( 'NONE',  ( -3.501826698183285735, 32.47146897220161321, 7.066576927953555298 ) ) ;
#2225=AXIS2_PLACEMENT_3D ( 'NONE', #4668, #2523, #3992 ) ;
#2226=ORIENTED_EDGE ( 'NONE', *, *, #2569, .T. ) ;
#2229=PLANE ( 'NONE',  #20 ) ;
#2237=CARTESIAN_POINT ( 'NONE',  ( 3.672134815396417284, 31.76998607164104627, 10.59780778022629200 ) ) ;
#2238=EDGE_CURVE ( 'NONE', #2608, #2276, #4654, .T. ) ;
#2239=CIRCLE ( 'NONE', #4693, 1.000000000000000888 ) ;
#2247=CARTESIAN_POINT ( 'NONE',  ( 3.707290417464801813, 34.32328140140740658, 10.50513240900691336 ) ) ;
#2251=EDGE_CURVE ( 'NONE', #3492, #1168, #608, .T. ) ;
#2252=ORIENTED_EDGE ( 'NONE', *, *, #2238, .F. ) ;
#2255=LINE ( 'NONE', #1196, #2114 ) ;
#2259=CARTESIAN_POINT ( 'NONE',  ( 3.469446951953614189E-15, 37.00000000000000000, 8.999999999999992895 ) ) ;
#2260=CIRCLE ( 'NONE', #222, 5.500000000000000000 ) ;
#2267=CARTESIAN_POINT ( 'NONE',  ( -3.877033663942010211, 31.25660811682476492, 7.985269980068073536 ) ) ;
#2268=CARTESIAN_POINT ( 'NONE',  ( 3.472015849686738598, 33.26730327278065147, 10.98645679572690348 ) ) ;
#2276=VERTEX_POINT ( 'NONE', #2098 ) ;
#2291=CARTESIAN_POINT ( 'NONE',  ( 3.948598437009898987, 34.89563602083902794, 8.348972239903947212 ) ) ;
#2295=ORIENTED_EDGE ( 'NONE', *, *, #1386, .F. ) ;
#2298=DIRECTION ( 'NONE',  ( -1.734723475976807094E-15, 0.000000000000000000, 1.000000000000000000 ) ) ;
#2301=DIRECTION ( 'NONE',  ( -0.000000000000000000, -1.000000000000000000, -0.000000000000000000 ) ) ;
#2303=CARTESIAN_POINT ( 'NONE',  ( -4.528983652092210654, 43.00000000000000000, 5.879373928346826261 ) ) ;
#2311=CIRCLE ( 'NONE', #4081, 1.000000000000000000 ) ;
#2313=CARTESIAN_POINT ( 'NONE',  ( 3.872084230669218918, 34.73127030857578745, 10.00969786038576714 ) ) ;
#2314=AXIS2_PLACEMENT_3D ( 'NONE', #2160, #1425, #5 ) ;
#2322=CARTESIAN_POINT ( 'NONE',  ( -4.528983652092209766, 37.00000000000000000, 5.879373928346827149 ) ) ;
#2325=VECTOR ( 'NONE', #2467, 1000.000000000000000 ) ;
#2330=STYLED_ITEM('',(#4729),#3033);
#2332=AXIS2_PLACEMENT_3D ( 'NONE', #120, #2651, #4116 ) ;
#2338=VERTEX_POINT ( 'NONE', #4293 ) ;
#2342=( NAMED_UNIT ( * ) PLANE_ANGLE_UNIT ( ) SI_UNIT ( $, .RADIAN. ) );
#2344=DIRECTION ( 'NONE',  ( 0.000000000000000000, 1.000000000000000000, 0.000000000000000000 ) ) ;
#2348=DIRECTION ( 'NONE',  ( 8.881784197001260212E-16, 0.000000000000000000, 1.000000000000000000 ) ) ;
#2350=ADVANCED_FACE ( 'NONE', ( #1693 ), #3145, .F. ) ;
#2355=EDGE_CURVE ( 'NONE', #1930, #525, #2763, .T. ) ;
#2359=AXIS2_PLACEMENT_3D ( 'NONE', #1364, #2466, #1385 ) ;
#2363=ORIENTED_EDGE ( 'NONE', *, *, #4242, .F. ) ;
#2366=DIRECTION ( 'NONE',  ( 0.000000000000000000, 0.000000000000000000, 1.000000000000000000 ) ) ;
#2375=AXIS2_PLACEMENT_3D ( 'NONE', #3819, #1254, #1672 ) ;
#2381=DIRECTION ( 'NONE',  ( 0.000000000000000000, 0.000000000000000000, 1.000000000000000000 ) ) ;
#2382=DIRECTION ( 'NONE',  ( 0.000000000000000000, 0.000000000000000000, 1.000000000000000000 ) ) ;
#2384=STYLED_ITEM ( 'NONE', ( #1641 ), #1996 ) ;
#2393=CYLINDRICAL_SURFACE ( 'NONE', #2535, 1.000000000000000000 ) ;
#2398=FACE_OUTER_BOUND ( 'NONE', #1615, .T. ) ;
#2402=CARTESIAN_POINT ( 'NONE',  ( 3.889087296525981063, 49.00000000000000000, 12.88908729652603746 ) ) ;
#2410=ORIENTED_EDGE ( 'NONE', *, *, #50, .T. ) ;
#2412=LINE ( 'NONE', #1400, #1232 ) ;
#2416=PRODUCT_DEFINITION_CONTEXT ( 'detailed design', #35, 'design' ) ;
#2423=EDGE_LOOP ( 'NONE', ( #3539, #3282, #304, #1635 ) ) ;
#2429=EDGE_CURVE ( 'NONE', #3445, #4670, #3484, .T. ) ;
#2436=VECTOR ( 'NONE', #4530, 1000.000000000000000 ) ;
#2441=DIRECTION ( 'NONE',  ( 0.000000000000000000, 0.000000000000000000, 1.000000000000000000 ) ) ;
#2462=CARTESIAN_POINT ( 'NONE',  ( 3.469446951953614189E-15, 43.00000000000000000, 8.999999999999992895 ) ) ;
#2466=DIRECTION ( 'NONE',  ( 0.000000000000000000, 1.000000000000000000, 0.000000000000000000 ) ) ;
#2467=DIRECTION ( 'NONE',  ( -0.000000000000000000, 1.000000000000000000, -0.000000000000000000 ) ) ;
#2470=AXIS2_PLACEMENT_3D ( 'NONE', #2462, #2117, #26 ) ;
#2475=EDGE_CURVE ( 'NONE', #4670, #3343, #3026, .T. ) ;
#2487=CIRCLE ( 'NONE', #4106, 4.000000000000000000 ) ;
#2499=EDGE_CURVE ( 'NONE', #4272, #1192, #2204, .T. ) ;
#2517=CYLINDRICAL_SURFACE ( 'NONE', #3800, 1.000000000000000000 ) ;
#2523=DIRECTION ( 'NONE',  ( 0.000000000000000000, 1.000000000000000000, 0.000000000000000000 ) ) ;
#2524=CARTESIAN_POINT ( 'NONE',  ( -4.528983652092254175, 43.00000000000000000, 12.12062607165309558 ) ) ;
#2527=CIRCLE ( 'NONE', #2225, 5.500000000000000000 ) ;
#2534=ORIENTED_EDGE ( 'NONE', *, *, #542, .T. ) ;
#2535=AXIS2_PLACEMENT_3D ( 'NONE', #3861, #605, #133 ) ;
#2544=CARTESIAN_POINT ( 'NONE',  ( -5.409090909090905619, 33.00000000000000000, 8.999999999999992895 ) ) ;
#2554=CARTESIAN_POINT ( 'NONE',  ( -3.672180636677252696, 31.77719734705737764, 7.412133430177195947 ) ) ;
#2559=ORIENTED_EDGE ( 'NONE', *, *, #2499, .F. ) ;
#2562=ADVANCED_FACE ( 'NONE', ( #530 ), #2612, .F. ) ;
#2567=ORIENTED_EDGE ( 'NONE', *, *, #1066, .T. ) ;
#2569=EDGE_CURVE ( 'NONE', #3374, #4356, #2255, .T. ) ;
#2573=CIRCLE ( 'NONE', #3564, 1.000000000000000000 ) ;
#2579=ORIENTED_EDGE ( 'NONE', *, *, #3271, .T. ) ;
#2583=ORIENTED_EDGE ( 'NONE', *, *, #253, .T. ) ;
#2586=EDGE_CURVE ( 'NONE', #3868, #1490, #2644, .T. ) ;
#2594=CARTESIAN_POINT ( 'NONE',  ( 0.9958591954639605115, 43.00000000000000000, 3.590909090909087276 ) ) ;
#2597=DIRECTION ( 'NONE',  ( 0.000000000000000000, 0.000000000000000000, 1.000000000000000000 ) ) ;
#2601=CYLINDRICAL_SURFACE ( 'NONE', #2842, 0.9999999999999991118 ) ;
#2605=EDGE_CURVE ( 'NONE', #377, #3402, #294, .T. ) ;
#2606=DIRECTION ( 'NONE',  ( -0.000000000000000000, -1.000000000000000000, -0.000000000000000000 ) ) ;
#2608=VERTEX_POINT ( 'NONE', #2710 ) ;
#2612=CYLINDRICAL_SURFACE ( 'NONE', #2723, 2.000000000000000888 ) ;
#2616=DIRECTION ( 'NONE',  ( -0.000000000000000000, -1.000000000000000000, -0.000000000000000000 ) ) ;
#2620=DIRECTION ( 'NONE',  ( -0.000000000000000000, 1.000000000000000000, 0.000000000000000000 ) ) ;
#2622=VECTOR ( 'NONE', #1420, 1000.000000000000000 ) ;
#2625=CARTESIAN_POINT ( 'NONE',  ( -3.999956176514747774, 34.99991235301547476, 8.865408859660240282 ) ) ;
#2626=CARTESIAN_POINT ( 'NONE',  ( 3.601840573626714281, 31.98585904651807965, 7.256529352857231885 ) ) ;
#2627=EDGE_LOOP ( 'NONE', ( #2295, #1954, #8, #881 ) ) ;
#2628=ORIENTED_EDGE ( 'NONE', *, *, #1556, .F. ) ;
#2630=CARTESIAN_POINT ( 'NONE',  ( -3.999885695961624243, 31.00022860814012660, 9.266511461428610374 ) ) ;
#2631=CARTESIAN_POINT ( 'NONE',  ( 3.464101615137757051, 33.13239633626785974, 10.99999999999999645 ) ) ;
#2632=EDGE_CURVE ( 'NONE', #4108, #213, #3327, .T. ) ;
#2634=ORIENTED_EDGE ( 'NONE', *, *, #696, .T. ) ;
#2638=UNCERTAINTY_MEASURE_WITH_UNIT (LENGTH_MEASURE( 1.000000000000000082E-05 ), #3790, 'distance_accuracy_value', 'NONE');
#2639=DIRECTION ( 'NONE',  ( 0.000000000000000000, 1.000000000000000000, 0.000000000000000000 ) ) ;
#2641=DIRECTION ( 'NONE',  ( 0.000000000000000000, -1.000000000000000000, 0.000000000000000000 ) ) ;
#2644=CIRCLE ( 'NONE', #1791, 5.500000000000000000 ) ;
#2649=ORIENTED_EDGE ( 'NONE', *, *, #215, .T. ) ;
#2651=DIRECTION ( 'NONE',  ( 0.000000000000000000, 1.000000000000000000, 0.000000000000000000 ) ) ;
#2654=ORIENTED_EDGE ( 'NONE', *, *, #3709, .F. ) ;
#2665=DIRECTION ( 'NONE',  ( 0.000000000000000000, 1.000000000000000000, 0.000000000000000000 ) ) ;
#2672=DIRECTION ( 'NONE',  ( 0.000000000000000000, 0.000000000000000000, 1.000000000000000000 ) ) ;
#2675=CARTESIAN_POINT ( 'NONE',  ( 3.501495480098620217, 33.52633409191729186, 10.93402018205975779 ) ) ;
#2678=EDGE_LOOP ( 'NONE', ( #3844, #2951 ) ) ;
#2682=CARTESIAN_POINT ( 'NONE',  ( -3.120626071653209710, 43.00000000000000000, 13.52898365209217246 ) ) ;
#2686=VERTEX_POINT ( 'NONE', #502 ) ;
#2687=CIRCLE ( 'NONE', #4224, 0.9999999999999995559 ) ;
#2694=AXIS2_PLACEMENT_3D ( 'NONE', #4505, #2301, #1248 ) ;
#2710=CARTESIAN_POINT ( 'NONE',  ( 3.469446951953614189E-15, 37.00000000000000000, 4.999999999999992006 ) ) ;
#2711=LINE ( 'NONE', #2682, #3810 ) ;
#2717=DIRECTION ( 'NONE',  ( -0.000000000000000000, -1.000000000000000000, -0.000000000000000000 ) ) ;
#2723=AXIS2_PLACEMENT_3D ( 'NONE', #813, #2973, #4500 ) ;
#2725=DIRECTION ( 'NONE',  ( 0.000000000000000000, 1.000000000000000000, 0.000000000000000000 ) ) ;
#2748=AXIS2_PLACEMENT_3D ( 'NONE', #2259, #2665, #4131 ) ;
#2757=ORIENTED_EDGE ( 'NONE', *, *, #583, .F. ) ;
#2758=DIRECTION ( 'NONE',  ( 0.000000000000000000, 1.000000000000000000, 0.000000000000000000 ) ) ;
#2760=( NAMED_UNIT ( * ) PLANE_ANGLE_UNIT ( ) SI_UNIT ( $, .RADIAN. ) );
#2762=DIRECTION ( 'NONE',  ( 0.000000000000000000, 1.000000000000000000, 0.000000000000000000 ) ) ;
#2763=LINE ( 'NONE', #653, #4506 ) ;
#2781=EDGE_CURVE ( 'NONE', #3119, #3995, #2260, .T. ) ;
#2784=DIRECTION ( 'NONE',  ( 0.000000000000000000, -1.000000000000000000, -0.000000000000000000 ) ) ;
#2789=CARTESIAN_POINT ( 'NONE',  ( 3.469446951953614189E-15, 43.00000000000000000, 4.999999999999992006 ) ) ;
#2793=CARTESIAN_POINT ( 'NONE',  ( -5.499999999999996447, 49.00000000000000000, 8.999999999999992895 ) ) ;
#2794=EDGE_CURVE ( 'NONE', #525, #2276, #2487, .T. ) ;
#2799=DIRECTION ( 'NONE',  ( 0.000000000000000000, 0.000000000000000000, -1.000000000000000000 ) ) ;
#2800=CIRCLE ( 'NONE', #4396, 0.9999999999999991118 ) ;
#2801=CARTESIAN_POINT ( 'NONE',  ( 5.409090909090911836, 37.00000000000000000, 9.995859195463930646 ) ) ;
#2803=ORIENTED_EDGE ( 'NONE', *, *, #3093, .T. ) ;
#2824=CARTESIAN_POINT ( 'NONE',  ( -3.948082828799468480, 34.89455565685986471, 8.346052798592715760 ) ) ;
#2827=ORIENTED_EDGE ( 'NONE', *, *, #538, .F. ) ;
#2840=PLANE ( 'NONE',  #264 ) ;
#2842=AXIS2_PLACEMENT_3D ( 'NONE', #439, #4440, #1581 ) ;
#2844=AXIS2_PLACEMENT_3D ( 'NONE', #139, #1578, #2597 ) ;
#2845=FACE_OUTER_BOUND ( 'NONE', #1068, .T. ) ;
#2851=DIRECTION ( 'NONE',  ( -0.000000000000000000, 1.000000000000000000, -0.000000000000000000 ) ) ;
#2859=LINE ( 'NONE', #293, #2325 ) ;
#2865=ADVANCED_FACE ( 'NONE', ( #670 ), #3562, .F. ) ;
#2870=CARTESIAN_POINT ( 'NONE',  ( -3.889087296526055226, 37.00000000000000000, 12.88908729652595753 ) ) ;
#2881=LINE ( 'NONE', #4629, #4638 ) ;
#2884=EDGE_CURVE ( 'NONE', #3374, #1902, #1136, .T. ) ;
#2888=AXIS2_PLACEMENT_3D ( 'NONE', #4597, #1341, #577 ) ;
#2894=ORIENTED_EDGE ( 'NONE', *, *, #3273, .F. ) ;
#2897=ADVANCED_FACE ( 'NONE', ( #1411 ), #3845, .T. ) ;
#2898=CARTESIAN_POINT ( 'NONE',  ( -3.672066530599461753, 31.77752803659710068, 10.58813356411692830 ) ) ;
#2901=ORIENTED_EDGE ( 'NONE', *, *, #4060, .F. ) ;
#2904=CIRCLE ( 'NONE', #852, 5.500000000000000000 ) ;
#2907=CARTESIAN_POINT ( 'NONE',  ( 3.464101615137757495, 33.00000000000000000, 6.999999999999991118 ) ) ;
#2915=DIRECTION ( 'NONE',  ( 0.000000000000000000, 1.000000000000000000, 0.000000000000000000 ) ) ;
#2916=CARTESIAN_POINT ( 'NONE',  ( -3.464101615137750834, 33.13465464847769937, 6.999999999999991118 ) ) ;
#2920=CIRCLE ( 'NONE', #2844, 1.000000000000000000 ) ;
#2921=DIRECTION ( 'NONE',  ( -0.000000000000000000, -1.000000000000000000, -0.000000000000000000 ) ) ;
#2924=ORIENTED_EDGE ( 'NONE', *, *, #2152, .F. ) ;
#2927=EDGE_CURVE ( 'NONE', #3868, #3995, #2800, .T. ) ;
#2928=AXIS2_PLACEMENT_3D ( 'NONE', #1780, #1712, #3957 ) ;
#2941=DIRECTION ( 'NONE',  ( 0.000000000000000000, 0.000000000000000000, 1.000000000000000000 ) ) ;
#2944=ORIENTED_EDGE ( 'NONE', *, *, #2499, .T. ) ;
#2946=CARTESIAN_POINT ( 'NONE',  ( -3.967498225428652159, 31.06568771763734560, 8.474567154859101947 ) ) ;
#2950=ORIENTED_EDGE ( 'NONE', *, *, #564, .F. ) ;
#2951=ORIENTED_EDGE ( 'NONE', *, *, #1011, .T. ) ;
#2952=DIRECTION ( 'NONE',  ( 0.000000000000000000, 1.000000000000000000, -0.000000000000000000 ) ) ;
#2964=CARTESIAN_POINT ( 'NONE',  ( -3.871991356174924181, 34.73106507380368413, 10.01005989714294842 ) ) ;
#2965=VERTEX_POINT ( 'NONE', #61 ) ;
#2967=CARTESIAN_POINT ( 'NONE',  ( 0.9958591954639605115, 49.00000000000000000, 3.590909090909087276 ) ) ;
#2972=UNCERTAINTY_MEASURE_WITH_UNIT (LENGTH_MEASURE( 1.000000000000000082E-05 ), #917, 'distance_accuracy_value', 'NONE');
#2973=DIRECTION ( 'NONE',  ( 1.000000000000000000, -0.000000000000000000, -0.000000000000000000 ) ) ;
#2980=DIRECTION ( 'NONE',  ( 0.000000000000000000, 0.000000000000000000, -1.000000000000000000 ) ) ;
#2983=EDGE_CURVE ( 'NONE', #834, #1543, #1433, .T. ) ;
#2990=CARTESIAN_POINT ( 'NONE',  ( -3.464101615137752166, 32.86760366373215447, 10.99999999999999822 ) ) ;
#2991=DIRECTION ( 'NONE',  ( 0.000000000000000000, -0.000000000000000000, 1.000000000000000000 ) ) ;
#2993=DIRECTION ( 'NONE',  ( 0.000000000000000000, 0.000000000000000000, 1.000000000000000000 ) ) ;
#2994=EDGE_LOOP ( 'NONE', ( #3252, #1422, #3567, #408 ) ) ;
#3004=VECTOR ( 'NONE', #2641, 1000.000000000000000 ) ;
#3006=CARTESIAN_POINT ( 'NONE',  ( 3.471741185006992136, 32.73575814869636957, 10.98693824102217853 ) ) ;
#3008=ADVANCED_FACE ( 'NONE', ( #1525 ), #1082, .F. ) ;
#3019=ORIENTED_EDGE ( 'NONE', *, *, #2927, .F. ) ;
#3026=CIRCLE ( 'NONE', #1732, 5.500000000000000000 ) ;
#3033=MANIFOLD_SOLID_BREP ( 'Cut-Extrude2', #1991 ) ;
#3035=CARTESIAN_POINT ( 'NONE',  ( -3.464101615137749057, 33.13263078466293621, 10.99999999999999289 ) ) ;
#3039=ORIENTED_EDGE ( 'NONE', *, *, #2355, .T. ) ;
#3040=AXIS2_PLACEMENT_3D ( 'NONE', #25, #2921, #760 ) ;
#3052=ORIENTED_EDGE ( 'NONE', *, *, #2213, .F. ) ;
#3055=DIRECTION ( 'NONE',  ( 0.000000000000000000, 1.000000000000000000, 0.000000000000000000 ) ) ;
#3061=CARTESIAN_POINT ( 'NONE',  ( 3.877033663942015984, 34.74339188317524219, 7.985269980068071760 ) ) ;
#3067=ORIENTED_EDGE ( 'NONE', *, *, #2238, .T. ) ;
#3076=AXIS2_PLACEMENT_3D ( 'NONE', #4011, #2190, #4388 ) ;
#3078=CARTESIAN_POINT ( 'NONE',  ( 3.469446951953614189E-15, 49.00000000000000000, 8.999999999999992895 ) ) ;
#3093=EDGE_CURVE ( 'NONE', #2276, #525, #3871, .T. ) ;
#3105=ORIENTED_EDGE ( 'NONE', *, *, #3093, .F. ) ;
#3108=ADVANCED_FACE ( 'NONE', ( #2398 ), #3767, .T. ) ;
#3115=DIRECTION ( 'NONE',  ( 0.000000000000000000, 1.000000000000000000, 0.000000000000000000 ) ) ;
#3118=ORIENTED_EDGE ( 'NONE', *, *, #2632, .T. ) ;
#3119=VERTEX_POINT ( 'NONE', #559 ) ;
#3123=DIRECTION ( 'NONE',  ( 0.000000000000000000, 1.000000000000000000, 0.000000000000000000 ) ) ;
#3130=ADVANCED_FACE ( 'NONE', ( #3797 ), #1624, .T. ) ;
#3141=DIRECTION ( 'NONE',  ( 0.000000000000000000, 0.000000000000000000, 1.000000000000000000 ) ) ;
#3144=CARTESIAN_POINT ( 'NONE',  ( 2.255140518769849223E-14, 49.00000000000000000, 3.499999999999992895 ) ) ;
#3145=CYLINDRICAL_SURFACE ( 'NONE', #1534, 1.000000000000000888 ) ;
#3149=CARTESIAN_POINT ( 'NONE',  ( 2.255140518769849223E-14, 37.00000000000000000, 3.499999999999992895 ) ) ;
#3152=DIRECTION ( 'NONE',  ( 0.000000000000000000, 0.000000000000000000, -1.000000000000000000 ) ) ;
#3164=ORIENTED_EDGE ( 'NONE', *, *, #1556, .T. ) ;
#3173=ORIENTED_EDGE ( 'NONE', *, *, #1240, .F. ) ;
#3181=CARTESIAN_POINT ( 'NONE',  ( -3.672900200782970526, 34.23223752615971449, 7.403954086897937437 ) ) ;
#3188=EDGE_CURVE ( 'NONE', #2608, #1930, #63, .T. ) ;
#3203=ORIENTED_EDGE ( 'NONE', *, *, #745, .F. ) ;
#3205=VECTOR ( 'NONE', #844, 1000.000000000000000 ) ;
#3207=EDGE_CURVE ( 'NONE', #3445, #3995, #2881, .T. ) ;
#3209=DIRECTION ( 'NONE',  ( -0.000000000000000000, -1.000000000000000000, -0.000000000000000000 ) ) ;
#3219=CARTESIAN_POINT ( 'NONE',  ( 4.000043395258034096, 30.99991320946996964, 9.131973577465631209 ) ) ;
#3235=DIRECTION ( 'NONE',  ( -1.000000000000000000, 0.000000000000000000, -3.469446951953614189E-15 ) ) ;
#3238=CARTESIAN_POINT ( 'NONE',  ( 3.469446951953614189E-15, 37.00000000000000000, 8.999999999999992895 ) ) ;
#3243=DIRECTION ( 'NONE',  ( 0.000000000000000000, 1.000000000000000000, 0.000000000000000000 ) ) ;
#3252=ORIENTED_EDGE ( 'NONE', *, *, #538, .T. ) ;
#3262=CARTESIAN_POINT ( 'NONE',  ( -3.889087296526001047, 34.17157287525380838, 5.110912703473974084 ) ) ;
#3265=CARTESIAN_POINT ( 'NONE',  ( 3.948285692887626652, 31.10501000327115761, 9.652966208173760165 ) ) ;
#3271=EDGE_CURVE ( 'NONE', #377, #2686, #2859, .T. ) ;
#3272=CARTESIAN_POINT ( 'NONE',  ( -0.9958591954639913757, 49.00000000000000000, 14.40909090909089230 ) ) ;
#3273=EDGE_CURVE ( 'NONE', #2091, #4272, #3952, .T. ) ;
#3274=ORIENTED_EDGE ( 'NONE', *, *, #613, .F. ) ;
#3275=ORIENTED_EDGE ( 'NONE', *, *, #2605, .F. ) ;
#3276=CARTESIAN_POINT ( 'NONE',  ( -3.606676218660104016, 31.99081763496160136, 7.268492701228250752 ) ) ;
#3282=ORIENTED_EDGE ( 'NONE', *, *, #3848, .T. ) ;
#3289=LINE ( 'NONE', #1478, #872 ) ;
#3294=CARTESIAN_POINT ( 'NONE',  ( 3.464101615137757495, 33.00000000000000000, 6.999999999999991118 ) ) ;
#3298=CARTESIAN_POINT ( 'NONE',  ( -4.000056596598882130, 30.99988680677069297, 8.869325943800758338 ) ) ;
#3304=ADVANCED_FACE ( 'NONE', ( #4493 ), #2517, .F. ) ;
#3315=CARTESIAN_POINT ( 'NONE',  ( 4.528983652092238188, 49.00000000000000000, 5.879373928346857348 ) ) ;
#3316=CARTESIAN_POINT ( 'NONE',  ( 2.255140518769849223E-14, 34.17157287525380838, 3.499999999999992895 ) ) ;
#3319=B_SPLINE_CURVE_WITH_KNOTS ( 'NONE', 3,
 ( #2154, #2916, #3993, #3534, #734, #1728, #3181, #4644, #1374, #2824, #1019, #4393, #2625, #116, #3671, #391, #4418, #1160, #2964, #4089, #825, #441, #3721, #2195, #1231, #1558, #3035, #1865 ),
 .UNSPECIFIED., .F., .F.,
 ( 4, 2, 2, 2, 2, 2, 2, 2, 2, 2, 2, 2, 2, 4 ),
 ( 0.000000000000000000, 0.0003975746136738172597, 0.0007951492273476345194, 0.001590298454695269689, 0.002385447682042904968, 0.002783022295716721956, 0.003180596909390539379, 0.003578171523064356801, 0.003975746136738173356, 0.004373320750411991212, 0.004770895364085809068, 0.005566044591433457790, 0.005963619205107282585, 0.006361193818781107380 ),
 .UNSPECIFIED. ) ;
#3322=AXIS2_PLACEMENT_3D ( 'NONE', #3411, #158, #1599 ) ;
#3327=CIRCLE ( 'NONE', #4549, 5.500000000000000000 ) ;
#3334=EDGE_CURVE ( 'NONE', #1199, #574, #963, .T. ) ;
#3338=CARTESIAN_POINT ( 'NONE',  ( -3.120626071653210154, 37.00000000000000000, 13.52898365209217246 ) ) ;
#3342=CARTESIAN_POINT ( 'NONE',  ( 0.9958591954638856825, 43.00000000000000000, 14.40909090909091361 ) ) ;
#3343=VERTEX_POINT ( 'NONE', #3703 ) ;
#3347=CARTESIAN_POINT ( 'NONE',  ( 5.409090909090912724, 49.00000000000000000, 8.004140804536053366 ) ) ;
#3356=CARTESIAN_POINT ( 'NONE',  ( 3.469446951953614189E-15, 49.00000000000000000, 8.999999999999992895 ) ) ;
#3358=ADVANCED_FACE ( 'NONE', ( #806 ), #4472, .T. ) ;
#3368=ORIENTED_EDGE ( 'NONE', *, *, #4269, .T. ) ;
#3369=CARTESIAN_POINT ( 'NONE',  ( -3.464101615137750390, 33.00000000000000000, 10.99999999999999467 ) ) ;
#3370=CARTESIAN_POINT ( 'NONE',  ( 3.464101615137757495, 33.13441662254499676, 6.999999999999990230 ) ) ;
#3371=CARTESIAN_POINT ( 'NONE',  ( 3.889087296525981063, 34.17157287525380838, 12.88908729652603746 ) ) ;
#3374=VERTEX_POINT ( 'NONE', #3347 ) ;
#3377=DIRECTION ( 'NONE',  ( 0.000000000000000000, 0.000000000000000000, 1.000000000000000000 ) ) ;
#3382=SHAPE_REPRESENTATION ( 'start button', ( #2928 ), #3388 ) ;
#3388=( GEOMETRIC_REPRESENTATION_CONTEXT ( 3 ) GLOBAL_UNCERTAINTY_ASSIGNED_CONTEXT ( ( #4455 ) ) GLOBAL_UNIT_ASSIGNED_CONTEXT ( ( #1961, #2342, #604 ) ) REPRESENTATION_CONTEXT ( 'NONE', 'WORKASPACE' ) );
#3395=EDGE_CURVE ( 'NONE', #1485, #377, #3702, .T. ) ;
#3402=VERTEX_POINT ( 'NONE', #851 ) ;
#3411=CARTESIAN_POINT ( 'NONE',  ( 3.469446951953614189E-15, 49.00000000000000000, 8.999999999999992895 ) ) ;
#3415=AXIS2_PLACEMENT_3D ( 'NONE', #889, #3123, #2051 ) ;
#3417=CARTESIAN_POINT ( 'NONE',  ( -3.889087296526001047, 49.00000000000000000, 5.110912703473974084 ) ) ;
#3420=DIRECTION ( 'NONE',  ( -0.000000000000000000, 1.000000000000000000, -0.000000000000000000 ) ) ;
#3424=ORIENTED_EDGE ( 'NONE', *, *, #3709, .T. ) ;
#3426=ORIENTED_EDGE ( 'NONE', *, *, #3888, .F. ) ;
#3439=CARTESIAN_POINT ( 'NONE',  ( 3.469446951953614189E-15, 37.00000000000000000, 8.999999999999992895 ) ) ;
#3443=CARTESIAN_POINT ( 'NONE',  ( -3.120626071653146649, 37.00000000000000000, 4.471016347907768029 ) ) ;
#3445=VERTEX_POINT ( 'NONE', #4235 ) ;
#3451=SHAPE_REPRESENTATION_RELATIONSHIP ( 'NONE' , 'NONE' ,  #3382, #1996 ) ;
#3459=DIRECTION ( 'NONE',  ( 0.000000000000000000, 0.000000000000000000, 1.000000000000000000 ) ) ;
#3464=DIRECTION ( 'NONE',  ( 0.000000000000000000, 1.000000000000000000, 0.000000000000000000 ) ) ;
#3466=AXIS2_PLACEMENT_3D ( 'NONE', #3439, #1678, #4611 ) ;
#3468=DIRECTION ( 'NONE',  ( -0.000000000000000000, -1.000000000000000000, -0.000000000000000000 ) ) ;
#3470=ORIENTED_EDGE ( 'NONE', *, *, #924, .F. ) ;
#3479=CARTESIAN_POINT ( 'NONE',  ( 5.409090909090912724, 43.00000000000000000, 9.995859195463930646 ) ) ;
#3484=CIRCLE ( 'NONE', #3866, 0.9999999999999991118 ) ;
#3486=CYLINDRICAL_SURFACE ( 'NONE', #870, 1.000000000000000000 ) ;
#3492=VERTEX_POINT ( 'NONE', #2801 ) ;
#3499=DIRECTION ( 'NONE',  ( -0.7071067811865484609, 0.000000000000000000, 0.7071067811865467956 ) ) ;
#3508=DIRECTION ( 'NONE',  ( 0.000000000000000000, 1.000000000000000000, 0.000000000000000000 ) ) ;
#3517=CARTESIAN_POINT ( 'NONE',  ( -4.528983652092254175, 49.00000000000000000, 12.12062607165309558 ) ) ;
#3523=CIRCLE ( 'NONE', #1467, 1.000000000000000000 ) ;
#3532=EDGE_CURVE ( 'NONE', #763, #460, #4329, .T. ) ;
#3534=CARTESIAN_POINT ( 'NONE',  ( -3.501309621998935917, 33.52503659006909942, 7.065645527993494213 ) ) ;
#3538=ORIENTED_EDGE ( 'NONE', *, *, #84, .T. ) ;
#3539=ORIENTED_EDGE ( 'NONE', *, *, #2605, .T. ) ;
#3550=CARTESIAN_POINT ( 'NONE',  ( 3.464101615137757495, 33.00000000000000000, 6.999999999999991118 ) ) ;
#3555=DIRECTION ( 'NONE',  ( -0.000000000000000000, 1.000000000000000000, 0.000000000000000000 ) ) ;
#3561=EDGE_CURVE ( 'NONE', #4272, #1877, #1022, .T. ) ;
#3562=CYLINDRICAL_SURFACE ( 'NONE', #3796, 0.9999999999999991118 ) ;
#3564=AXIS2_PLACEMENT_3D ( 'NONE', #1322, #2762, #3499 ) ;
#3566=LINE ( 'NONE', #1051, #277 ) ;
#3567=ORIENTED_EDGE ( 'NONE', *, *, #4242, .T. ) ;
#3574=CARTESIAN_POINT ( 'NONE',  ( -5.409090909090905619, 49.00000000000000000, 8.004140804536053366 ) ) ;
#3579=FACE_BOUND ( 'NONE', #1659, .T. ) ;
#3580=CYLINDRICAL_SURFACE ( 'NONE', #4439, 1.000000000000000000 ) ;
#3590=DIRECTION ( 'NONE',  ( 0.000000000000000000, 0.000000000000000000, 1.000000000000000000 ) ) ;
#3610=LINE ( 'NONE', #717, #1833 ) ;
#3611=FACE_BOUND ( 'NONE', #2093, .T. ) ;
#3617=DIRECTION ( 'NONE',  ( 0.000000000000000000, 0.000000000000000000, 1.000000000000000000 ) ) ;
#3619=CARTESIAN_POINT ( 'NONE',  ( 3.464101615137757495, 33.00000000000000000, 10.99999999999999467 ) ) ;
#3620=LINE ( 'NONE', #359, #342 ) ;
#3623=ADVANCED_FACE ( 'NONE', ( #4690 ), #1459, .F. ) ;
#3631=ORIENTED_EDGE ( 'NONE', *, *, #2794, .F. ) ;
#3632=CARTESIAN_POINT ( 'NONE',  ( -3.523178763948781711, 32.34692174699498679, 7.105158153061386983 ) ) ;
#3634=DIRECTION ( 'NONE',  ( 0.000000000000000000, 0.000000000000000000, -1.000000000000000000 ) ) ;
#3636=EDGE_CURVE ( 'NONE', #1877, #3492, #3748, .T. ) ;
#3637=( GEOMETRIC_REPRESENTATION_CONTEXT ( 3 ) GLOBAL_UNCERTAINTY_ASSIGNED_CONTEXT ( ( #2972 ) ) GLOBAL_UNIT_ASSIGNED_CONTEXT ( ( #917, #967, #4226 ) ) REPRESENTATION_CONTEXT ( 'NONE', 'WORKASPACE' ) );
#3641=FACE_OUTER_BOUND ( 'NONE', #1492, .T. ) ;
#3645=CARTESIAN_POINT ( 'NONE',  ( 3.775090262067429148, 31.49720376393407761, 10.32592777499123926 ) ) ;
#3653=ORIENTED_EDGE ( 'NONE', *, *, #1240, .T. ) ;
#3654=FACE_OUTER_BOUND ( 'NONE', #3672, .T. ) ;
#3660=ORIENTED_EDGE ( 'NONE', *, *, #2429, .F. ) ;
#3671=CARTESIAN_POINT ( 'NONE',  ( -3.993226401463528141, 34.98654878845945859, 9.266623410949812012 ) ) ;
#3672=EDGE_LOOP ( 'NONE', ( #2634, #4594, #2182, #2226 ) ) ;
#3674=AXIS2_PLACEMENT_3D ( 'NONE', #3149, #3867, #2348 ) ;
#3676=CARTESIAN_POINT ( 'NONE',  ( -3.464101615137750390, 33.00000000000000000, 6.999999999999991118 ) ) ;
#3678=CARTESIAN_POINT ( 'NONE',  ( 4.528983652092195555, 49.00000000000000000, 12.12062607165318973 ) ) ;
#3680=EDGE_LOOP ( 'NONE', ( #4041, #53, #3, #1612 ) ) ;
#3689=CIRCLE ( 'NONE', #1862, 1.000000000000000888 ) ;
#3697=VERTEX_POINT ( 'NONE', #1437 ) ;
#3702=CIRCLE ( 'NONE', #2332, 5.500000000000000000 ) ;
#3703=CARTESIAN_POINT ( 'NONE',  ( -4.528983652092253287, 37.00000000000000000, 12.12062607165309558 ) ) ;
#3708=ORIENTED_EDGE ( 'NONE', *, *, #3532, .T. ) ;
#3709=EDGE_CURVE ( 'NONE', #2338, #1543, #2527, .T. ) ;
#3714=ORIENTED_EDGE ( 'NONE', *, *, #4060, .T. ) ;
#3719=CARTESIAN_POINT ( 'NONE',  ( 3.959305671612554781E-15, 37.00000000000000000, 12.99999999999999289 ) ) ;
#3721=CARTESIAN_POINT ( 'NONE',  ( -3.601048973789305219, 34.01100974488973350, 10.74504312029988107 ) ) ;
#3722=AXIS2_PLACEMENT_3D ( 'NONE', #1075, #2180, #3634 ) ;
#3725=CARTESIAN_POINT ( 'NONE',  ( -3.810302108970980761, 31.40405275936838336, 7.767247897850001692 ) ) ;
#3731=ORIENTED_EDGE ( 'NONE', *, *, #2586, .F. ) ;
#3735=CARTESIAN_POINT ( 'NONE',  ( 3.120626071653185285, 43.00000000000000000, 4.471016347907789346 ) ) ;
#3737=ADVANCED_FACE ( 'NONE', ( #1373 ), #3580, .F. ) ;
#3740=ADVANCED_FACE ( 'NONE', ( #1532 ), #2601, .F. ) ;
#3744=AXIS2_PLACEMENT_3D ( 'NONE', #3144, #986, #3235 ) ;
#3748=CIRCLE ( 'NONE', #4221, 5.500000000000000000 ) ;
#3751=CARTESIAN_POINT ( 'NONE',  ( 3.889087296526035242, 49.00000000000000000, 6.110912703473999841 ) ) ;
#3767=CYLINDRICAL_SURFACE ( 'NONE', #3322, 5.500000000000000000 ) ;
#3778=DIRECTION ( 'NONE',  ( -0.7071067811865484609, 0.000000000000000000, 0.7071067811865467956 ) ) ;
#3779=B_SPLINE_CURVE_WITH_KNOTS ( 'NONE', 3,
 ( #3369, #2990, #4043, #445, #73, #4447, #47, #2898, #4351, #1463, #1487, #3996, #1163, #2179, #2630, #3298, #1186, #2946, #4397, #2267, #3725, #785, #2554, #3276, #738, #3632, #2221, #1120, #4372, #3676 ),
 .UNSPECIFIED., .F., .F.,
 ( 4, 2, 2, 2, 2, 2, 2, 2, 2, 2, 2, 2, 2, 2, 4 ),
 ( 0.006361193818781107380, 0.006758065648931978198, 0.007154937479082849015, 0.007551809309233719833, 0.007948681139384591518, 0.008345552969535447591, 0.008742424799686305398, 0.009536168459988021012, 0.009933040290138880554, 0.01032991212028973836, 0.01112365578059145224, 0.01152052761074230137, 0.01191739944089315051, 0.01231427127104400138, 0.01271114310119485051 ),
 .UNSPECIFIED. ) ;
#3781=CARTESIAN_POINT ( 'NONE',  ( 4.000056596598889236, 35.00011319322931769, 8.869325943800760115 ) ) ;
#3790=( LENGTH_UNIT ( ) NAMED_UNIT ( * ) SI_UNIT ( .MILLI., .METRE. ) );
#3796=AXIS2_PLACEMENT_3D ( 'NONE', #306, #3926, #1013 ) ;
#3797=FACE_OUTER_BOUND ( 'NONE', #1267, .T. ) ;
#3800=AXIS2_PLACEMENT_3D ( 'NONE', #3262, #3420, #98 ) ;
#3810=VECTOR ( 'NONE', #2784, 1000.000000000000000 ) ;
#3819=CARTESIAN_POINT ( 'NONE',  ( 3.469446951953614189E-15, 37.00000000000000000, 8.999999999999992895 ) ) ;
#3820=CIRCLE ( 'NONE', #16, 1.000000000000000000 ) ;
#3821=ORIENTED_EDGE ( 'NONE', *, *, #925, .F. ) ;
#3830=ORIENTED_EDGE ( 'NONE', *, *, #1129, .T. ) ;
#3844=ORIENTED_EDGE ( 'NONE', *, *, #3188, .T. ) ;
#3845=CYLINDRICAL_SURFACE ( 'NONE', #1432, 5.500000000000000000 ) ;
#3848=EDGE_CURVE ( 'NONE', #3402, #3855, #1557, .T. ) ;
#3855=VERTEX_POINT ( 'NONE', #415 ) ;
#3856=ORIENTED_EDGE ( 'NONE', *, *, #3207, .F. ) ;
#3861=CARTESIAN_POINT ( 'NONE',  ( 2.255140518769849223E-14, 34.17157287525380838, 3.499999999999992895 ) ) ;
#3863=ADVANCED_FACE ( 'NONE', ( #182 ), #3486, .F. ) ;
#3866=AXIS2_PLACEMENT_3D ( 'NONE', #1450, #2185, #1078 ) ;
#3867=DIRECTION ( 'NONE',  ( -0.000000000000000000, -1.000000000000000000, -0.000000000000000000 ) ) ;
#3868=VERTEX_POINT ( 'NONE', #922 ) ;
#3871=CIRCLE ( 'NONE', #4483, 4.000000000000000000 ) ;
#3875=CARTESIAN_POINT ( 'NONE',  ( 4.528983652092238188, 43.00000000000000000, 5.879373928346857348 ) ) ;
#3881=FACE_OUTER_BOUND ( 'NONE', #599, .T. ) ;
#3888=EDGE_CURVE ( 'NONE', #1185, #1192, #3523, .T. ) ;
#3902=CARTESIAN_POINT ( 'NONE',  ( 3.889087296526035242, 34.17157287525380838, 5.110912703473999841 ) ) ;
#3910=CIRCLE ( 'NONE', #2375, 5.500000000000000000 ) ;
#3919=DIRECTION ( 'NONE',  ( 0.000000000000000000, 0.000000000000000000, 1.000000000000000000 ) ) ;
#3920=DIRECTION ( 'NONE',  ( -0.000000000000000000, -1.000000000000000000, -0.000000000000000000 ) ) ;
#3926=DIRECTION ( 'NONE',  ( -0.000000000000000000, 1.000000000000000000, -0.000000000000000000 ) ) ;
#3942=CARTESIAN_POINT ( 'NONE',  ( 3.501309621998943467, 32.47496340993090058, 7.065645527993491548 ) ) ;
#3943=CARTESIAN_POINT ( 'NONE',  ( 0.9958591954639605115, 37.00000000000000000, 3.590909090909087276 ) ) ;
#3952=CIRCLE ( 'NONE', #1505, 5.500000000000000000 ) ;
#3957=DIRECTION ( 'NONE',  ( 1.000000000000000000, 0.000000000000000000, 0.000000000000000000 ) ) ;
#3959=ORIENTED_EDGE ( 'NONE', *, *, #2983, .T. ) ;
#3963=DIRECTION ( 'NONE',  ( 0.000000000000000000, 1.000000000000000000, 0.000000000000000000 ) ) ;
#3965=AXIS2_PLACEMENT_3D ( 'NONE', #448, #1540, #2993 ) ;
#3966=DIRECTION ( 'NONE',  ( -0.000000000000000000, 1.000000000000000000, -0.000000000000000000 ) ) ;
#3971=CARTESIAN_POINT ( 'NONE',  ( 3.959305671612554781E-15, 25.00000000000000000, 12.99999999999999289 ) ) ;
#3979=ORIENTED_EDGE ( 'NONE', *, *, #4098, .F. ) ;
#3983=CARTESIAN_POINT ( 'NONE',  ( 3.672180636677260246, 34.22280265294261170, 7.412133430177196836 ) ) ;
#3991=ADVANCED_FACE ( 'NONE', ( #709, #2172 ), #2840, .F. ) ;
#3992=DIRECTION ( 'NONE',  ( 0.000000000000000000, 0.000000000000000000, 1.000000000000000000 ) ) ;
#3993=CARTESIAN_POINT ( 'NONE',  ( -3.471963499745391868, 33.26650496313073546, 7.013453814050720325 ) ) ;
#3994=EDGE_LOOP ( 'NONE', ( #1568, #4452, #3067, #2803 ) ) ;
#3995=VERTEX_POINT ( 'NONE', #3574 ) ;
#3996=CARTESIAN_POINT ( 'NONE',  ( -3.872084230669213145, 31.26872969142421255, 10.00969786038576714 ) ) ;
#4011=CARTESIAN_POINT ( 'NONE',  ( 3.469446951953614189E-15, 49.00000000000000000, 8.999999999999992895 ) ) ;
#4017=CARTESIAN_POINT ( 'NONE',  ( -3.120626071653209266, 49.00000000000000000, 13.52898365209217246 ) ) ;
#4037=EDGE_CURVE ( 'NONE', #574, #1199, #939, .T. ) ;
#4041=ORIENTED_EDGE ( 'NONE', *, *, #2781, .F. ) ;
#4043=CARTESIAN_POINT ( 'NONE',  ( -3.472015849686731048, 32.73269672721935564, 10.98645679572690170 ) ) ;
#4055=ORIENTED_EDGE ( 'NONE', *, *, #3636, .F. ) ;
#4060=EDGE_CURVE ( 'NONE', #1922, #1485, #2920, .T. ) ;
#4065=CARTESIAN_POINT ( 'NONE',  ( -5.377642775528101993E-14, 37.00000000000000000, 14.49999999999999289 ) ) ;
#4081=AXIS2_PLACEMENT_3D ( 'NONE', #3417, #3464, #3778 ) ;
#4088=DIRECTION ( 'NONE',  ( -0.000000000000000000, 1.000000000000000000, -0.000000000000000000 ) ) ;
#4089=CARTESIAN_POINT ( 'NONE',  ( -3.809422024637061810, 34.58617949464730401, 10.22508852591142059 ) ) ;
#4091=ORIENTED_EDGE ( 'NONE', *, *, #2475, .F. ) ;
#4094=CARTESIAN_POINT ( 'NONE',  ( 3.472185852622990065, 33.26949845712274367, 7.013837769849709858 ) ) ;
#4096=DIRECTION ( 'NONE',  ( -0.000000000000000000, -1.000000000000000000, 0.000000000000000000 ) ) ;
#4098=EDGE_CURVE ( 'NONE', #213, #460, #3289, .T. ) ;
#4106=AXIS2_PLACEMENT_3D ( 'NONE', #1340, #936, #2366 ) ;
#4108=VERTEX_POINT ( 'NONE', #3338 ) ;
#4113=LINE ( 'NONE', #141, #589 ) ;
#4116=DIRECTION ( 'NONE',  ( 0.000000000000000000, 0.000000000000000000, 1.000000000000000000 ) ) ;
#4119=EDGE_CURVE ( 'NONE', #468, #460, #2010, .T. ) ;
#4131=DIRECTION ( 'NONE',  ( 0.000000000000000000, 0.000000000000000000, 1.000000000000000000 ) ) ;
#4138=AXIS2_PLACEMENT_3D ( 'NONE', #666, #3555, #3919 ) ;
#4140=CARTESIAN_POINT ( 'NONE',  ( 3.775946040281031646, 34.50493851269693124, 10.32350191120197813 ) ) ;
#4141=CARTESIAN_POINT ( 'NONE',  ( 4.528983652092195555, 43.00000000000000000, 12.12062607165318973 ) ) ;
#4146=ORIENTED_EDGE ( 'NONE', *, *, #1264, .T. ) ;
#4153=FACE_OUTER_BOUND ( 'NONE', #1447, .T. ) ;
#4161=VECTOR ( 'NONE', #1533, 1000.000000000000000 ) ;
#4164=CIRCLE ( 'NONE', #3722, 0.9999999999999991118 ) ;
#4182=CARTESIAN_POINT ( 'NONE',  ( 3.469446951953614189E-15, 49.00000000000000000, 8.999999999999992895 ) ) ;
#4184=AXIS2_PLACEMENT_3D ( 'NONE', #2544, #341, #2980 ) ;
#4195=DIRECTION ( 'NONE',  ( -0.7071067811865437980, 0.000000000000000000, -0.7071067811865512365 ) ) ;
#4202=CYLINDRICAL_SURFACE ( 'NONE', #2694, 5.500000000000000000 ) ;
#4216=DIRECTION ( 'NONE',  ( -0.000000000000000000, 1.000000000000000000, -0.000000000000000000 ) ) ;
#4218=ORIENTED_EDGE ( 'NONE', *, *, #3334, .T. ) ;
#4221=AXIS2_PLACEMENT_3D ( 'NONE', #1818, #2915, #4368 ) ;
#4224=AXIS2_PLACEMENT_3D ( 'NONE', #203, #3055, #1302 ) ;
#4226=( NAMED_UNIT ( * ) SI_UNIT ( $, .STERADIAN. ) SOLID_ANGLE_UNIT ( ) );
#4235=CARTESIAN_POINT ( 'NONE',  ( -5.409090909090905619, 37.00000000000000000, 8.004140804536053366 ) ) ;
#4242=EDGE_CURVE ( 'NONE', #468, #1490, #2687, .T. ) ;
#4251=CARTESIAN_POINT ( 'NONE',  ( 3.469446951953614189E-15, 49.00000000000000000, 8.999999999999992895 ) ) ;
#4260=ORIENTED_EDGE ( 'NONE', *, *, #3561, .T. ) ;
#4267=DIRECTION ( 'NONE',  ( -0.000000000000000000, 1.000000000000000000, 0.000000000000000000 ) ) ;
#4269=EDGE_CURVE ( 'NONE', #2965, #834, #3910, .T. ) ;
#4272=VERTEX_POINT ( 'NONE', #159 ) ;
#4285=ORIENTED_EDGE ( 'NONE', *, *, #3636, .T. ) ;
#4291=ORIENTED_EDGE ( 'NONE', *, *, #543, .T. ) ;
#4293=CARTESIAN_POINT ( 'NONE',  ( 3.120626071653185285, 49.00000000000000000, 4.471016347907789346 ) ) ;
#4299=CARTESIAN_POINT ( 'NONE',  ( 3.469446951953614189E-15, 37.00000000000000000, 8.999999999999992895 ) ) ;
#4304=CYLINDRICAL_SURFACE ( 'NONE', #4348, 4.000000000000000000 ) ;
#4317=DIRECTION ( 'NONE',  ( 0.000000000000000000, 0.000000000000000000, -1.000000000000000000 ) ) ;
#4320=CARTESIAN_POINT ( 'NONE',  ( 3.471963499745398973, 32.73349503686927164, 7.013453814050719437 ) ) ;
#4328=ORIENTED_EDGE ( 'NONE', *, *, #1440, .F. ) ;
#4329=CIRCLE ( 'NONE', #291, 1.000000000000000000 ) ;
#4348=AXIS2_PLACEMENT_3D ( 'NONE', #1044, #4642, #2799 ) ;
#4351=CARTESIAN_POINT ( 'NONE',  ( -3.707290417464794707, 31.67671859859259698, 10.50513240900691159 ) ) ;
#4352=EDGE_CURVE ( 'NONE', #834, #1922, #412, .T. ) ;
#4355=ORIENTED_EDGE ( 'NONE', *, *, #711, .F. ) ;
#4356=VERTEX_POINT ( 'NONE', #560 ) ;
#4359=CARTESIAN_POINT ( 'NONE',  ( 3.900821110013157789, 34.79398413074517293, 9.893616917921782772 ) ) ;
#4368=DIRECTION ( 'NONE',  ( 0.000000000000000000, 0.000000000000000000, 1.000000000000000000 ) ) ;
#4370=ORIENTED_EDGE ( 'NONE', *, *, #564, .T. ) ;
#4372=CARTESIAN_POINT ( 'NONE',  ( -3.464101615137749501, 32.86558337745499614, 6.999999999999988454 ) ) ;
#4388=DIRECTION ( 'NONE',  ( 0.000000000000000000, 0.000000000000000000, 1.000000000000000000 ) ) ;
#4393=CARTESIAN_POINT ( 'NONE',  ( -3.993269581196945417, 34.98663585528726117, 8.733908321742497094 ) ) ;
#4396=AXIS2_PLACEMENT_3D ( 'NONE', #2793, #273, #1721 ) ;
#4397=CARTESIAN_POINT ( 'NONE',  ( -3.948598437009891882, 31.10436397916096496, 8.348972239903947212 ) ) ;
#4406=CARTESIAN_POINT ( 'NONE',  ( 3.469446951953614189E-15, 25.00000000000000000, 8.999999999999992895 ) ) ;
#4418=CARTESIAN_POINT ( 'NONE',  ( -3.948285692887619991, 34.89498999672885304, 9.652966208173760165 ) ) ;
#4419=ORIENTED_EDGE ( 'NONE', *, *, #2632, .F. ) ;
#4421=CARTESIAN_POINT ( 'NONE',  ( 3.469446951953614189E-15, 49.00000000000000000, 8.999999999999992895 ) ) ;
#4432=CARTESIAN_POINT ( 'NONE',  ( 3.889087296526035242, 37.00000000000000000, 5.110912703473999841 ) ) ;
#4435=CARTESIAN_POINT ( 'NONE',  ( 3.464101615137757495, 33.00000000000000000, 10.99999999999999467 ) ) ;
#4437=EDGE_CURVE ( 'NONE', #3868, #4670, #3620, .T. ) ;
#4439=AXIS2_PLACEMENT_3D ( 'NONE', #3316, #873, #2941 ) ;
#4440=DIRECTION ( 'NONE',  ( -0.000000000000000000, 1.000000000000000000, -0.000000000000000000 ) ) ;
#4447=CARTESIAN_POINT ( 'NONE',  ( -3.575798854573970509, 32.10535367473890744, 10.79358726550605851 ) ) ;
#4450=CYLINDRICAL_SURFACE ( 'NONE', #2130, 1.000000000000000888 ) ;
#4451=ORIENTED_EDGE ( 'NONE', *, *, #1871, .F. ) ;
#4452=ORIENTED_EDGE ( 'NONE', *, *, #3188, .F. ) ;
#4455=UNCERTAINTY_MEASURE_WITH_UNIT (LENGTH_MEASURE( 1.000000000000000082E-05 ), #1961, 'distance_accuracy_value', 'NONE');
#4462=CARTESIAN_POINT ( 'NONE',  ( -0.9958591954639161026, 43.00000000000000000, 3.590909090909080170 ) ) ;
#4472=PLANE ( 'NONE',  #2108 ) ;
#4475=LINE ( 'NONE', #4141, #307 ) ;
#4477=ORIENTED_EDGE ( 'NONE', *, *, #4037, .T. ) ;
#4483=AXIS2_PLACEMENT_3D ( 'NONE', #1965, #2007, #3459 ) ;
#4489=AXIS2_PLACEMENT_3D ( 'NONE', #286, #671, #4672 ) ;
#4493=FACE_OUTER_BOUND ( 'NONE', #2423, .T. ) ;
#4494=PRODUCT_DEFINITION_SHAPE ( 'NONE', 'NONE',  #487 ) ;
#4495=CARTESIAN_POINT ( 'NONE',  ( 3.464101615137757495, 33.00000000000000000, 10.99999999999999467 ) ) ;
#4500=DIRECTION ( 'NONE',  ( 0.000000000000000000, 0.000000000000000000, -1.000000000000000000 ) ) ;
#4505=CARTESIAN_POINT ( 'NONE',  ( 3.469446951953614189E-15, 49.00000000000000000, 8.999999999999992895 ) ) ;
#4506=VECTOR ( 'NONE', #4553, 1000.000000000000000 ) ;
#4507=CARTESIAN_POINT ( 'NONE',  ( 3.469446951953614189E-15, 49.00000000000000000, 8.999999999999992895 ) ) ;
#4516=CARTESIAN_POINT ( 'NONE',  ( 3.810302108970986978, 34.59594724063161664, 7.767247897849999028 ) ) ;
#4525=CARTESIAN_POINT ( 'NONE',  ( -3.464101615137750390, 33.00000000000000000, 10.99999999999999467 ) ) ;
#4527=( NAMED_UNIT ( * ) SI_UNIT ( $, .STERADIAN. ) SOLID_ANGLE_UNIT ( ) );
#4530=DIRECTION ( 'NONE',  ( 0.000000000000000000, -1.000000000000000000, 0.000000000000000000 ) ) ;
#4539=CARTESIAN_POINT ( 'NONE',  ( -5.377642775528101993E-14, 49.00000000000000000, 14.49999999999999289 ) ) ;
#4549=AXIS2_PLACEMENT_3D ( 'NONE', #1220, #2639, #3377 ) ;
#4551=EDGE_CURVE ( 'NONE', #2338, #2965, #1198, .T. ) ;
#4553=DIRECTION ( 'NONE',  ( -0.000000000000000000, -1.000000000000000000, -0.000000000000000000 ) ) ;
#4559=ORIENTED_EDGE ( 'NONE', *, *, #4269, .F. ) ;
#4562=ADVANCED_FACE ( 'NONE', ( #940 ), #4202, .T. ) ;
#4563=CIRCLE ( 'NONE', #3415, 0.9999999999999997780 ) ;
#4564=DIRECTION ( 'NONE',  ( 0.000000000000000000, 0.000000000000000000, 1.000000000000000000 ) ) ;
#4570=ORIENTED_EDGE ( 'NONE', *, *, #2142, .F. ) ;
#4579=CARTESIAN_POINT ( 'NONE',  ( -5.377642775528101993E-14, 34.17157287525380838, 14.49999999999999289 ) ) ;
#4585=DIRECTION ( 'NONE',  ( 0.7071067811865536790, 0.000000000000000000, -0.7071067811865415775 ) ) ;
#4592=DIRECTION ( 'NONE',  ( -0.000000000000000000, 1.000000000000000000, -0.000000000000000000 ) ) ;
#4594=ORIENTED_EDGE ( 'NONE', *, *, #250, .T. ) ;
#4597=CARTESIAN_POINT ( 'NONE',  ( 3.469446951953614189E-15, 49.00000000000000000, 8.999999999999992895 ) ) ;
#4609=CIRCLE ( 'NONE', #1792, 1.000000000000000000 ) ;
#4611=DIRECTION ( 'NONE',  ( 0.000000000000000000, 0.000000000000000000, 1.000000000000000000 ) ) ;
#4613=CIRCLE ( 'NONE', #2314, 4.000000000000000000 ) ;
#4629=CARTESIAN_POINT ( 'NONE',  ( -5.409090909090905619, 43.00000000000000000, 8.004140804536053366 ) ) ;
#4638=VECTOR ( 'NONE', #1387, 1000.000000000000000 ) ;
#4640=AXIS2_PLACEMENT_3D ( 'NONE', #4507, #1251, #581 ) ;
#4642=DIRECTION ( 'NONE',  ( -0.000000000000000000, -1.000000000000000000, -0.000000000000000000 ) ) ;
#4644=CARTESIAN_POINT ( 'NONE',  ( -3.809991693235069476, 34.59507057476615444, 7.766500207085086593 ) ) ;
#4650=CYLINDRICAL_SURFACE ( 'NONE', #1784, 1.000000000000000000 ) ;
#4653=ADVANCED_FACE ( 'NONE', ( #964 ), #2393, .F. ) ;
#4654=LINE ( 'NONE', #2789, #941 ) ;
#4662=CARTESIAN_POINT ( 'NONE',  ( 3.523144759583864527, 32.34704090027811674, 7.105089090000585195 ) ) ;
#4668=CARTESIAN_POINT ( 'NONE',  ( 3.469446951953614189E-15, 49.00000000000000000, 8.999999999999992895 ) ) ;
#4670=VERTEX_POINT ( 'NONE', #4673 ) ;
#4671=ORIENTED_EDGE ( 'NONE', *, *, #4551, .F. ) ;
#4672=DIRECTION ( 'NONE',  ( 0.000000000000000000, 0.000000000000000000, -1.000000000000000000 ) ) ;
#4673=CARTESIAN_POINT ( 'NONE',  ( -5.409090909090905619, 37.00000000000000000, 9.995859195463932423 ) ) ;
#4683=EDGE_CURVE ( 'NONE', #3492, #4356, #1943, .T. ) ;
#4684=DIRECTION ( 'NONE',  ( 0.000000000000000000, 1.000000000000000000, 0.000000000000000000 ) ) ;
#4687=CARTESIAN_POINT ( 'NONE',  ( 3.993226401463535247, 31.01345121154055207, 9.266623410949817341 ) ) ;
#4690=FACE_OUTER_BOUND ( 'NONE', #2994, .T. ) ;
#4691=DIRECTION ( 'NONE',  ( 0.000000000000000000, 0.000000000000000000, 1.000000000000000000 ) ) ;
#4693=AXIS2_PLACEMENT_3D ( 'NONE', #2870, #3920, #4691 ) ;
#4695=ORIENTED_EDGE ( 'NONE', *, *, #3395, .F. ) ;
#4698=DIRECTION ( 'NONE',  ( 0.000000000000000000, 0.000000000000000000, 1.000000000000000000 ) ) ;
#4700=ADVANCED_FACE ( 'NONE', ( #3881 ), #4650, .F. ) ;
#4701=EDGE_LOOP ( 'NONE', ( #1293, #4559, #3470, #4451, #51, #188, #4055, #1774, #2894, #2950, #4419, #2827, #4091, #3660, #942, #1637, #3275, #4695, #2901 ) ) ;
#4723=COLOUR_RGB('Light Blue',0.38,0.62,0.78);
#4724=FILL_AREA_STYLE_COLOUR('',#4723);
#4725=FILL_AREA_STYLE('',(#4724));
#4726=SURFACE_STYLE_FILL_AREA(#4725);
#4727=SURFACE_SIDE_STYLE('',(#4726));
#4728=SURFACE_STYLE_USAGE(.BOTH.,#4727);
#4729=PRESENTATION_STYLE_ASSIGNMENT((#4728));
ENDSEC;
END-ISO-10303-21;
